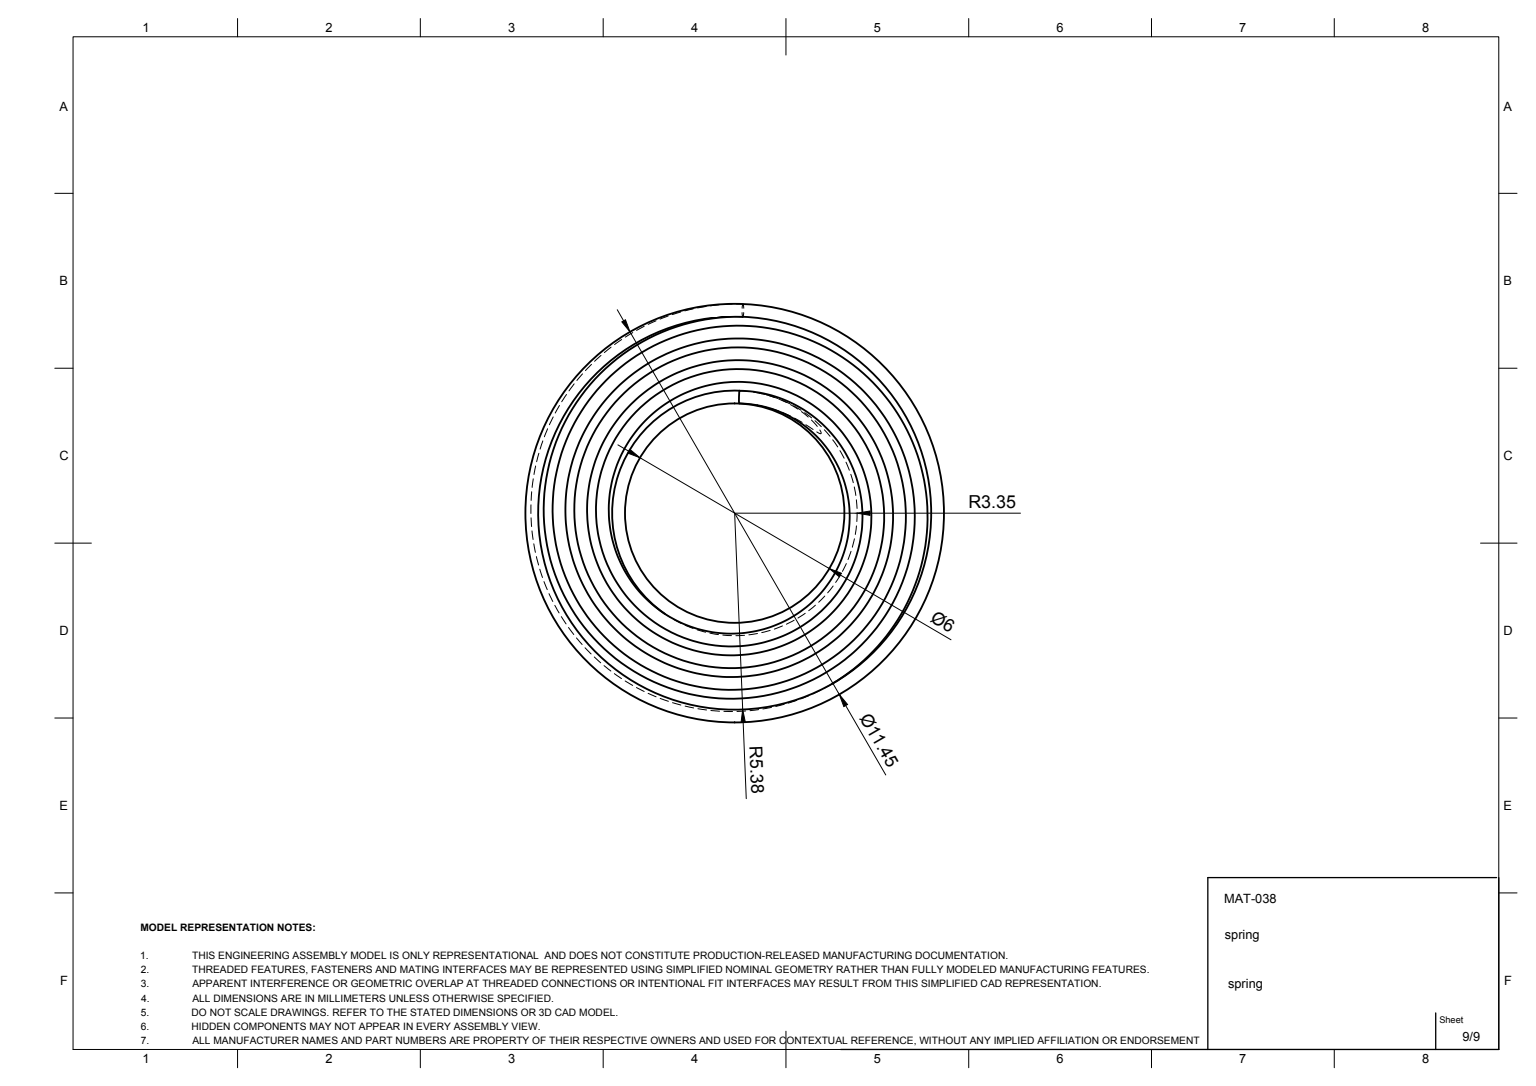
ISO-10303-21;
HEADER;
/* Generated by software containing ST-Developer
 * from STEP Tools, Inc. (www.steptools.com) 
 */

FILE_DESCRIPTION(
/* description */ ('STEP AP214'),
/* implementation_level */ '2;1');

FILE_NAME(
/* name */ 'Spring.step',
/* time_stamp */ '2026-11-14T21:32:33-08:00',
/* author */ (''),
/* organization */ (''),
/* preprocessor_version */ 'ST-DEVELOPER v20.2',
/* originating_system */ 'Autodesk Translation Framework v15.17.0.0',
/* authorisation */ '');

FILE_SCHEMA (('AUTOMOTIVE_DESIGN { 1 0 10303 214 3 1 1 }'));
ENDSEC;

DATA;
#10=MECHANICAL_DESIGN_GEOMETRIC_PRESENTATION_REPRESENTATION('',(#185,#186),#10551);
#47=(
BOUNDED_SURFACE()
B_SPLINE_SURFACE(3,3,((#8436,#8437,#8438,#8439,#8440,#8441,#8442,#8443,
#8444,#8445,#8446,#8447,#8448,#8449,#8450,#8451,#8452,#8453,#8454,#8455,
#8456,#8457,#8458,#8459,#8460,#8461,#8462,#8463,#8464,#8465,#8466,#8467,
#8468,#8469,#8470,#8471,#8472,#8473,#8474,#8475,#8476,#8477,#8478,#8479,
#8480,#8481,#8482,#8483,#8484,#8485,#8486,#8487,#8488,#8489,#8490,#8491,
#8492,#8493,#8494,#8495,#8496,#8497,#8498,#8499,#8500,#8501,#8502,#8503,
#8504,#8505,#8506,#8507,#8508,#8509,#8510,#8511,#8512,#8513,#8514,#8515,
#8516,#8517,#8518,#8519,#8520,#8521,#8522,#8523,#8524,#8525,#8526,#8527,
#8528,#8529,#8530,#8531,#8532,#8533,#8534,#8535,#8536,#8537,#8538,#8539,
#8540,#8541,#8542,#8543,#8544,#8545,#8546,#8547,#8548,#8549,#8550,#8551,
#8552,#8553,#8554,#8555,#8556,#8557,#8558,#8559,#8560,#8561,#8562,#8563,
#8564,#8565),(#8566,#8567,#8568,#8569,#8570,#8571,#8572,#8573,#8574,#8575,
#8576,#8577,#8578,#8579,#8580,#8581,#8582,#8583,#8584,#8585,#8586,#8587,
#8588,#8589,#8590,#8591,#8592,#8593,#8594,#8595,#8596,#8597,#8598,#8599,
#8600,#8601,#8602,#8603,#8604,#8605,#8606,#8607,#8608,#8609,#8610,#8611,
#8612,#8613,#8614,#8615,#8616,#8617,#8618,#8619,#8620,#8621,#8622,#8623,
#8624,#8625,#8626,#8627,#8628,#8629,#8630,#8631,#8632,#8633,#8634,#8635,
#8636,#8637,#8638,#8639,#8640,#8641,#8642,#8643,#8644,#8645,#8646,#8647,
#8648,#8649,#8650,#8651,#8652,#8653,#8654,#8655,#8656,#8657,#8658,#8659,
#8660,#8661,#8662,#8663,#8664,#8665,#8666,#8667,#8668,#8669,#8670,#8671,
#8672,#8673,#8674,#8675,#8676,#8677,#8678,#8679,#8680,#8681,#8682,#8683,
#8684,#8685,#8686,#8687,#8688,#8689,#8690,#8691,#8692,#8693,#8694,#8695),
(#8696,#8697,#8698,#8699,#8700,#8701,#8702,#8703,#8704,#8705,#8706,#8707,
#8708,#8709,#8710,#8711,#8712,#8713,#8714,#8715,#8716,#8717,#8718,#8719,
#8720,#8721,#8722,#8723,#8724,#8725,#8726,#8727,#8728,#8729,#8730,#8731,
#8732,#8733,#8734,#8735,#8736,#8737,#8738,#8739,#8740,#8741,#8742,#8743,
#8744,#8745,#8746,#8747,#8748,#8749,#8750,#8751,#8752,#8753,#8754,#8755,
#8756,#8757,#8758,#8759,#8760,#8761,#8762,#8763,#8764,#8765,#8766,#8767,
#8768,#8769,#8770,#8771,#8772,#8773,#8774,#8775,#8776,#8777,#8778,#8779,
#8780,#8781,#8782,#8783,#8784,#8785,#8786,#8787,#8788,#8789,#8790,#8791,
#8792,#8793,#8794,#8795,#8796,#8797,#8798,#8799,#8800,#8801,#8802,#8803,
#8804,#8805,#8806,#8807,#8808,#8809,#8810,#8811,#8812,#8813,#8814,#8815,
#8816,#8817,#8818,#8819,#8820,#8821,#8822,#8823,#8824,#8825),(#8826,#8827,
#8828,#8829,#8830,#8831,#8832,#8833,#8834,#8835,#8836,#8837,#8838,#8839,
#8840,#8841,#8842,#8843,#8844,#8845,#8846,#8847,#8848,#8849,#8850,#8851,
#8852,#8853,#8854,#8855,#8856,#8857,#8858,#8859,#8860,#8861,#8862,#8863,
#8864,#8865,#8866,#8867,#8868,#8869,#8870,#8871,#8872,#8873,#8874,#8875,
#8876,#8877,#8878,#8879,#8880,#8881,#8882,#8883,#8884,#8885,#8886,#8887,
#8888,#8889,#8890,#8891,#8892,#8893,#8894,#8895,#8896,#8897,#8898,#8899,
#8900,#8901,#8902,#8903,#8904,#8905,#8906,#8907,#8908,#8909,#8910,#8911,
#8912,#8913,#8914,#8915,#8916,#8917,#8918,#8919,#8920,#8921,#8922,#8923,
#8924,#8925,#8926,#8927,#8928,#8929,#8930,#8931,#8932,#8933,#8934,#8935,
#8936,#8937,#8938,#8939,#8940,#8941,#8942,#8943,#8944,#8945,#8946,#8947,
#8948,#8949,#8950,#8951,#8952,#8953,#8954,#8955),(#8956,#8957,#8958,#8959,
#8960,#8961,#8962,#8963,#8964,#8965,#8966,#8967,#8968,#8969,#8970,#8971,
#8972,#8973,#8974,#8975,#8976,#8977,#8978,#8979,#8980,#8981,#8982,#8983,
#8984,#8985,#8986,#8987,#8988,#8989,#8990,#8991,#8992,#8993,#8994,#8995,
#8996,#8997,#8998,#8999,#9000,#9001,#9002,#9003,#9004,#9005,#9006,#9007,
#9008,#9009,#9010,#9011,#9012,#9013,#9014,#9015,#9016,#9017,#9018,#9019,
#9020,#9021,#9022,#9023,#9024,#9025,#9026,#9027,#9028,#9029,#9030,#9031,
#9032,#9033,#9034,#9035,#9036,#9037,#9038,#9039,#9040,#9041,#9042,#9043,
#9044,#9045,#9046,#9047,#9048,#9049,#9050,#9051,#9052,#9053,#9054,#9055,
#9056,#9057,#9058,#9059,#9060,#9061,#9062,#9063,#9064,#9065,#9066,#9067,
#9068,#9069,#9070,#9071,#9072,#9073,#9074,#9075,#9076,#9077,#9078,#9079,
#9080,#9081,#9082,#9083,#9084,#9085),(#9086,#9087,#9088,#9089,#9090,#9091,
#9092,#9093,#9094,#9095,#9096,#9097,#9098,#9099,#9100,#9101,#9102,#9103,
#9104,#9105,#9106,#9107,#9108,#9109,#9110,#9111,#9112,#9113,#9114,#9115,
#9116,#9117,#9118,#9119,#9120,#9121,#9122,#9123,#9124,#9125,#9126,#9127,
#9128,#9129,#9130,#9131,#9132,#9133,#9134,#9135,#9136,#9137,#9138,#9139,
#9140,#9141,#9142,#9143,#9144,#9145,#9146,#9147,#9148,#9149,#9150,#9151,
#9152,#9153,#9154,#9155,#9156,#9157,#9158,#9159,#9160,#9161,#9162,#9163,
#9164,#9165,#9166,#9167,#9168,#9169,#9170,#9171,#9172,#9173,#9174,#9175,
#9176,#9177,#9178,#9179,#9180,#9181,#9182,#9183,#9184,#9185,#9186,#9187,
#9188,#9189,#9190,#9191,#9192,#9193,#9194,#9195,#9196,#9197,#9198,#9199,
#9200,#9201,#9202,#9203,#9204,#9205,#9206,#9207,#9208,#9209,#9210,#9211,
#9212,#9213,#9214,#9215),(#9216,#9217,#9218,#9219,#9220,#9221,#9222,#9223,
#9224,#9225,#9226,#9227,#9228,#9229,#9230,#9231,#9232,#9233,#9234,#9235,
#9236,#9237,#9238,#9239,#9240,#9241,#9242,#9243,#9244,#9245,#9246,#9247,
#9248,#9249,#9250,#9251,#9252,#9253,#9254,#9255,#9256,#9257,#9258,#9259,
#9260,#9261,#9262,#9263,#9264,#9265,#9266,#9267,#9268,#9269,#9270,#9271,
#9272,#9273,#9274,#9275,#9276,#9277,#9278,#9279,#9280,#9281,#9282,#9283,
#9284,#9285,#9286,#9287,#9288,#9289,#9290,#9291,#9292,#9293,#9294,#9295,
#9296,#9297,#9298,#9299,#9300,#9301,#9302,#9303,#9304,#9305,#9306,#9307,
#9308,#9309,#9310,#9311,#9312,#9313,#9314,#9315,#9316,#9317,#9318,#9319,
#9320,#9321,#9322,#9323,#9324,#9325,#9326,#9327,#9328,#9329,#9330,#9331,
#9332,#9333,#9334,#9335,#9336,#9337,#9338,#9339,#9340,#9341,#9342,#9343,
#9344,#9345)),.UNSPECIFIED.,.T.,.F.,.F.)
B_SPLINE_SURFACE_WITH_KNOTS((4,3,4),(4,2,2,2,2,2,2,2,2,2,2,2,2,2,2,2,2,
2,2,2,2,2,2,2,2,2,2,2,2,2,2,2,2,2,2,2,2,2,2,2,2,2,2,2,2,2,2,2,2,2,2,2,2,
2,2,2,2,2,2,2,2,2,2,2,4),(0.,0.5,1.),(-1.6716721247158E-5,0.015625,0.03125,
0.046875,0.0625,0.078125,0.09375,0.109375,0.125,0.140625,0.15625,0.171875,
0.1875,0.203125,0.21875,0.234375,0.25,0.265625,0.28125,0.296875,0.3125,
0.328125,0.34375,0.359375,0.375,0.390625,0.40625,0.421875,0.4375,0.453125,
0.46875,0.484375,0.5,0.515625,0.53125,0.546875,0.5625,0.578125,0.59375,
0.609375,0.625,0.640625,0.65625,0.671875,0.6875,0.703125,0.71875,0.734375,
0.75,0.765625,0.78125,0.796875,0.8125,0.828125,0.84375,0.859375,0.875,0.890625,
0.90625,0.921875,0.9375,0.953125,0.96875,0.984375,1.),.UNSPECIFIED.)
GEOMETRIC_REPRESENTATION_ITEM()
RATIONAL_B_SPLINE_SURFACE(((1.,1.,1.,1.,1.,1.,1.,1.,1.,1.,1.,1.,1.,1.,1.,
1.,1.,1.,1.,1.,1.,1.,1.,1.,1.,1.,1.,1.,1.,1.,1.,1.,1.,1.,1.,1.,1.,1.,1.,
1.,1.,1.,1.,1.,1.,1.,1.,1.,1.,1.,1.,1.,1.,1.,1.,1.,1.,1.,1.,1.,1.,1.,1.,
1.,1.,1.,1.,1.,1.,1.,1.,1.,1.,1.,1.,1.,1.,1.,1.,1.,1.,1.,1.,1.,1.,1.,1.,
1.,1.,1.,1.,1.,1.,1.,1.,1.,1.,1.,1.,1.,1.,1.,1.,1.,1.,1.,1.,1.,1.,1.,1.,
1.,1.,1.,1.,1.,1.,1.,1.,1.,1.,1.,1.,1.,1.,1.,1.,1.,1.,1.),(0.333333333333334,
0.333333333333333,0.333333333333333,0.333333333333333,0.333333333333333,
0.333333333333333,0.333333333333333,0.333333333333333,0.333333333333333,
0.333333333333333,0.333333333333333,0.333333333333333,0.333333333333333,
0.333333333333333,0.333333333333333,0.333333333333333,0.333333333333333,
0.333333333333333,0.333333333333333,0.333333333333333,0.333333333333333,
0.333333333333333,0.333333333333333,0.333333333333333,0.333333333333333,
0.333333333333333,0.333333333333333,0.333333333333333,0.333333333333333,
0.333333333333333,0.333333333333333,0.333333333333333,0.333333333333333,
0.333333333333333,0.333333333333333,0.333333333333333,0.333333333333333,
0.333333333333333,0.333333333333333,0.333333333333333,0.333333333333333,
0.333333333333333,0.333333333333333,0.333333333333333,0.333333333333333,
0.333333333333333,0.333333333333333,0.333333333333333,0.333333333333333,
0.333333333333333,0.333333333333333,0.333333333333333,0.333333333333333,
0.333333333333333,0.333333333333333,0.333333333333333,0.333333333333333,
0.333333333333333,0.333333333333333,0.333333333333333,0.333333333333333,
0.333333333333333,0.333333333333333,0.333333333333333,0.333333333333333,
0.333333333333333,0.333333333333333,0.333333333333333,0.333333333333333,
0.333333333333333,0.333333333333333,0.333333333333333,0.333333333333333,
0.333333333333333,0.333333333333333,0.333333333333333,0.333333333333333,
0.333333333333333,0.333333333333333,0.333333333333333,0.333333333333333,
0.333333333333333,0.333333333333333,0.333333333333333,0.333333333333333,
0.333333333333333,0.333333333333333,0.333333333333333,0.333333333333333,
0.333333333333333,0.333333333333333,0.333333333333333,0.333333333333333,
0.333333333333333,0.333333333333333,0.333333333333333,0.333333333333333,
0.333333333333333,0.333333333333333,0.333333333333333,0.333333333333333,
0.333333333333333,0.333333333333333,0.333333333333333,0.333333333333333,
0.333333333333333,0.333333333333333,0.333333333333333,0.333333333333333,
0.333333333333333,0.333333333333333,0.333333333333333,0.333333333333333,
0.333333333333333,0.333333333333333,0.333333333333333,0.333333333333333,
0.333333333333333,0.333333333333333,0.333333333333333,0.333333333333333,
0.333333333333333,0.333333333333333,0.333333333333333,0.333333333333333,
0.333333333333333,0.333333333333333,0.333333333333333,0.333333333333333,
0.333333333333333),(0.333333333333334,0.333333333333333,0.333333333333333,
0.333333333333333,0.333333333333333,0.333333333333333,0.333333333333333,
0.333333333333333,0.333333333333333,0.333333333333333,0.333333333333333,
0.333333333333333,0.333333333333333,0.333333333333333,0.333333333333333,
0.333333333333333,0.333333333333333,0.333333333333333,0.333333333333333,
0.333333333333333,0.333333333333333,0.333333333333333,0.333333333333333,
0.333333333333333,0.333333333333333,0.333333333333333,0.333333333333333,
0.333333333333333,0.333333333333333,0.333333333333333,0.333333333333333,
0.333333333333333,0.333333333333333,0.333333333333333,0.333333333333333,
0.333333333333333,0.333333333333333,0.333333333333333,0.333333333333333,
0.333333333333333,0.333333333333333,0.333333333333333,0.333333333333333,
0.333333333333333,0.333333333333333,0.333333333333333,0.333333333333333,
0.333333333333333,0.333333333333333,0.333333333333333,0.333333333333333,
0.333333333333333,0.333333333333333,0.333333333333333,0.333333333333333,
0.333333333333333,0.333333333333333,0.333333333333333,0.333333333333333,
0.333333333333333,0.333333333333333,0.333333333333333,0.333333333333333,
0.333333333333333,0.333333333333333,0.333333333333333,0.333333333333333,
0.333333333333333,0.333333333333333,0.333333333333333,0.333333333333333,
0.333333333333333,0.333333333333333,0.333333333333333,0.333333333333333,
0.333333333333333,0.333333333333333,0.333333333333333,0.333333333333333,
0.333333333333333,0.333333333333333,0.333333333333333,0.333333333333333,
0.333333333333333,0.333333333333333,0.333333333333333,0.333333333333333,
0.333333333333333,0.333333333333333,0.333333333333333,0.333333333333333,
0.333333333333333,0.333333333333333,0.333333333333333,0.333333333333333,
0.333333333333333,0.333333333333333,0.333333333333333,0.333333333333333,
0.333333333333333,0.333333333333333,0.333333333333333,0.333333333333333,
0.333333333333333,0.333333333333333,0.333333333333333,0.333333333333333,
0.333333333333333,0.333333333333333,0.333333333333333,0.333333333333333,
0.333333333333333,0.333333333333333,0.333333333333333,0.333333333333333,
0.333333333333333,0.333333333333333,0.333333333333333,0.333333333333333,
0.333333333333333,0.333333333333333,0.333333333333333,0.333333333333333,
0.333333333333333,0.333333333333333,0.333333333333333,0.333333333333333,
0.333333333333333,0.333333333333333,0.333333333333333),(1.,1.,1.,1.,1.,
1.,1.,1.,1.,1.,1.,1.,1.,1.,1.,1.,1.,1.,1.,1.,1.,1.,1.,1.,1.,1.,1.,1.,1.,
1.,1.,1.,1.,1.,1.,1.,1.,1.,1.,1.,1.,1.,1.,1.,1.,1.,1.,1.,1.,1.,1.,1.,1.,
1.,1.,1.,1.,1.,1.,1.,1.,1.,1.,1.,1.,1.,1.,1.,1.,1.,1.,1.,1.,1.,1.,1.,1.,
1.,1.,1.,1.,1.,1.,1.,1.,1.,1.,1.,1.,1.,1.,1.,1.,1.,1.,1.,1.,1.,1.,1.,1.,
1.,1.,1.,1.,1.,1.,1.,1.,1.,1.,1.,1.,1.,1.,1.,1.,1.,1.,1.,1.,1.,1.,1.,1.,
1.,1.,1.,1.,1.),(0.333333333333334,0.333333333333333,0.333333333333333,
0.333333333333333,0.333333333333333,0.333333333333333,0.333333333333333,
0.333333333333333,0.333333333333333,0.333333333333333,0.333333333333333,
0.333333333333333,0.333333333333333,0.333333333333333,0.333333333333333,
0.333333333333333,0.333333333333333,0.333333333333333,0.333333333333333,
0.333333333333333,0.333333333333333,0.333333333333333,0.333333333333333,
0.333333333333333,0.333333333333333,0.333333333333333,0.333333333333333,
0.333333333333333,0.333333333333333,0.333333333333333,0.333333333333333,
0.333333333333333,0.333333333333333,0.333333333333333,0.333333333333333,
0.333333333333333,0.333333333333333,0.333333333333333,0.333333333333333,
0.333333333333333,0.333333333333333,0.333333333333333,0.333333333333333,
0.333333333333333,0.333333333333333,0.333333333333333,0.333333333333333,
0.333333333333333,0.333333333333333,0.333333333333333,0.333333333333333,
0.333333333333333,0.333333333333333,0.333333333333333,0.333333333333333,
0.333333333333333,0.333333333333333,0.333333333333333,0.333333333333333,
0.333333333333333,0.333333333333333,0.333333333333333,0.333333333333333,
0.333333333333333,0.333333333333333,0.333333333333333,0.333333333333333,
0.333333333333333,0.333333333333333,0.333333333333333,0.333333333333333,
0.333333333333333,0.333333333333333,0.333333333333333,0.333333333333333,
0.333333333333333,0.333333333333333,0.333333333333333,0.333333333333333,
0.333333333333333,0.333333333333333,0.333333333333333,0.333333333333333,
0.333333333333333,0.333333333333333,0.333333333333333,0.333333333333333,
0.333333333333333,0.333333333333333,0.333333333333333,0.333333333333333,
0.333333333333333,0.333333333333333,0.333333333333333,0.333333333333333,
0.333333333333333,0.333333333333333,0.333333333333333,0.333333333333333,
0.333333333333333,0.333333333333333,0.333333333333333,0.333333333333333,
0.333333333333333,0.333333333333333,0.333333333333333,0.333333333333333,
0.333333333333333,0.333333333333333,0.333333333333333,0.333333333333333,
0.333333333333333,0.333333333333333,0.333333333333333,0.333333333333333,
0.333333333333333,0.333333333333333,0.333333333333333,0.333333333333333,
0.333333333333333,0.333333333333333,0.333333333333333,0.333333333333333,
0.333333333333333,0.333333333333333,0.333333333333333,0.333333333333333,
0.333333333333333,0.333333333333333,0.333333333333333),(0.333333333333334,
0.333333333333333,0.333333333333333,0.333333333333333,0.333333333333333,
0.333333333333333,0.333333333333333,0.333333333333333,0.333333333333333,
0.333333333333333,0.333333333333333,0.333333333333333,0.333333333333333,
0.333333333333333,0.333333333333333,0.333333333333333,0.333333333333333,
0.333333333333333,0.333333333333333,0.333333333333333,0.333333333333333,
0.333333333333333,0.333333333333333,0.333333333333333,0.333333333333333,
0.333333333333333,0.333333333333333,0.333333333333333,0.333333333333333,
0.333333333333333,0.333333333333333,0.333333333333333,0.333333333333333,
0.333333333333333,0.333333333333333,0.333333333333333,0.333333333333333,
0.333333333333333,0.333333333333333,0.333333333333333,0.333333333333333,
0.333333333333333,0.333333333333333,0.333333333333333,0.333333333333333,
0.333333333333333,0.333333333333333,0.333333333333333,0.333333333333333,
0.333333333333333,0.333333333333333,0.333333333333333,0.333333333333333,
0.333333333333333,0.333333333333333,0.333333333333333,0.333333333333333,
0.333333333333333,0.333333333333333,0.333333333333333,0.333333333333333,
0.333333333333333,0.333333333333333,0.333333333333333,0.333333333333333,
0.333333333333333,0.333333333333333,0.333333333333333,0.333333333333333,
0.333333333333333,0.333333333333333,0.333333333333333,0.333333333333333,
0.333333333333333,0.333333333333333,0.333333333333333,0.333333333333333,
0.333333333333333,0.333333333333333,0.333333333333333,0.333333333333333,
0.333333333333333,0.333333333333333,0.333333333333333,0.333333333333333,
0.333333333333333,0.333333333333333,0.333333333333333,0.333333333333333,
0.333333333333333,0.333333333333333,0.333333333333333,0.333333333333333,
0.333333333333333,0.333333333333333,0.333333333333333,0.333333333333333,
0.333333333333333,0.333333333333333,0.333333333333333,0.333333333333333,
0.333333333333333,0.333333333333333,0.333333333333333,0.333333333333333,
0.333333333333333,0.333333333333333,0.333333333333333,0.333333333333333,
0.333333333333333,0.333333333333333,0.333333333333333,0.333333333333333,
0.333333333333333,0.333333333333333,0.333333333333333,0.333333333333333,
0.333333333333333,0.333333333333333,0.333333333333333,0.333333333333333,
0.333333333333333,0.333333333333333,0.333333333333333,0.333333333333333,
0.333333333333333,0.333333333333333,0.333333333333333,0.333333333333333,
0.333333333333333),(1.,1.,1.,1.,1.,1.,1.,1.,1.,1.,1.,1.,1.,1.,1.,1.,1.,
1.,1.,1.,1.,1.,1.,1.,1.,1.,1.,1.,1.,1.,1.,1.,1.,1.,1.,1.,1.,1.,1.,1.,1.,
1.,1.,1.,1.,1.,1.,1.,1.,1.,1.,1.,1.,1.,1.,1.,1.,1.,1.,1.,1.,1.,1.,1.,1.,
1.,1.,1.,1.,1.,1.,1.,1.,1.,1.,1.,1.,1.,1.,1.,1.,1.,1.,1.,1.,1.,1.,1.,1.,
1.,1.,1.,1.,1.,1.,1.,1.,1.,1.,1.,1.,1.,1.,1.,1.,1.,1.,1.,1.,1.,1.,1.,1.,
1.,1.,1.,1.,1.,1.,1.,1.,1.,1.,1.,1.,1.,1.,1.,1.,1.)))
REPRESENTATION_ITEM('')
SURFACE()
);
#48=(
BOUNDED_SURFACE()
B_SPLINE_SURFACE(3,3,((#9609,#9610,#9611,#9612,#9613,#9614,#9615,#9616,
#9617,#9618,#9619,#9620,#9621,#9622,#9623,#9624,#9625,#9626,#9627,#9628,
#9629,#9630,#9631,#9632,#9633,#9634,#9635,#9636,#9637,#9638,#9639,#9640,
#9641,#9642,#9643,#9644,#9645,#9646,#9647,#9648,#9649,#9650,#9651,#9652,
#9653,#9654,#9655,#9656,#9657,#9658,#9659,#9660,#9661,#9662,#9663,#9664,
#9665,#9666,#9667,#9668,#9669,#9670,#9671,#9672,#9673,#9674,#9675,#9676,
#9677,#9678,#9679,#9680,#9681,#9682,#9683,#9684,#9685,#9686,#9687,#9688,
#9689,#9690,#9691,#9692,#9693,#9694,#9695,#9696,#9697,#9698,#9699,#9700,
#9701,#9702,#9703,#9704,#9705,#9706,#9707,#9708,#9709,#9710,#9711,#9712,
#9713,#9714,#9715,#9716,#9717,#9718,#9719,#9720,#9721,#9722,#9723,#9724,
#9725,#9726,#9727,#9728,#9729,#9730,#9731,#9732,#9733,#9734,#9735,#9736,
#9737,#9738),(#9739,#9740,#9741,#9742,#9743,#9744,#9745,#9746,#9747,#9748,
#9749,#9750,#9751,#9752,#9753,#9754,#9755,#9756,#9757,#9758,#9759,#9760,
#9761,#9762,#9763,#9764,#9765,#9766,#9767,#9768,#9769,#9770,#9771,#9772,
#9773,#9774,#9775,#9776,#9777,#9778,#9779,#9780,#9781,#9782,#9783,#9784,
#9785,#9786,#9787,#9788,#9789,#9790,#9791,#9792,#9793,#9794,#9795,#9796,
#9797,#9798,#9799,#9800,#9801,#9802,#9803,#9804,#9805,#9806,#9807,#9808,
#9809,#9810,#9811,#9812,#9813,#9814,#9815,#9816,#9817,#9818,#9819,#9820,
#9821,#9822,#9823,#9824,#9825,#9826,#9827,#9828,#9829,#9830,#9831,#9832,
#9833,#9834,#9835,#9836,#9837,#9838,#9839,#9840,#9841,#9842,#9843,#9844,
#9845,#9846,#9847,#9848,#9849,#9850,#9851,#9852,#9853,#9854,#9855,#9856,
#9857,#9858,#9859,#9860,#9861,#9862,#9863,#9864,#9865,#9866,#9867,#9868),
(#9869,#9870,#9871,#9872,#9873,#9874,#9875,#9876,#9877,#9878,#9879,#9880,
#9881,#9882,#9883,#9884,#9885,#9886,#9887,#9888,#9889,#9890,#9891,#9892,
#9893,#9894,#9895,#9896,#9897,#9898,#9899,#9900,#9901,#9902,#9903,#9904,
#9905,#9906,#9907,#9908,#9909,#9910,#9911,#9912,#9913,#9914,#9915,#9916,
#9917,#9918,#9919,#9920,#9921,#9922,#9923,#9924,#9925,#9926,#9927,#9928,
#9929,#9930,#9931,#9932,#9933,#9934,#9935,#9936,#9937,#9938,#9939,#9940,
#9941,#9942,#9943,#9944,#9945,#9946,#9947,#9948,#9949,#9950,#9951,#9952,
#9953,#9954,#9955,#9956,#9957,#9958,#9959,#9960,#9961,#9962,#9963,#9964,
#9965,#9966,#9967,#9968,#9969,#9970,#9971,#9972,#9973,#9974,#9975,#9976,
#9977,#9978,#9979,#9980,#9981,#9982,#9983,#9984,#9985,#9986,#9987,#9988,
#9989,#9990,#9991,#9992,#9993,#9994,#9995,#9996,#9997,#9998),(#9999,#10000,
#10001,#10002,#10003,#10004,#10005,#10006,#10007,#10008,#10009,#10010,#10011,
#10012,#10013,#10014,#10015,#10016,#10017,#10018,#10019,#10020,#10021,#10022,
#10023,#10024,#10025,#10026,#10027,#10028,#10029,#10030,#10031,#10032,#10033,
#10034,#10035,#10036,#10037,#10038,#10039,#10040,#10041,#10042,#10043,#10044,
#10045,#10046,#10047,#10048,#10049,#10050,#10051,#10052,#10053,#10054,#10055,
#10056,#10057,#10058,#10059,#10060,#10061,#10062,#10063,#10064,#10065,#10066,
#10067,#10068,#10069,#10070,#10071,#10072,#10073,#10074,#10075,#10076,#10077,
#10078,#10079,#10080,#10081,#10082,#10083,#10084,#10085,#10086,#10087,#10088,
#10089,#10090,#10091,#10092,#10093,#10094,#10095,#10096,#10097,#10098,#10099,
#10100,#10101,#10102,#10103,#10104,#10105,#10106,#10107,#10108,#10109,#10110,
#10111,#10112,#10113,#10114,#10115,#10116,#10117,#10118,#10119,#10120,#10121,
#10122,#10123,#10124,#10125,#10126,#10127,#10128),(#10129,#10130,#10131,
#10132,#10133,#10134,#10135,#10136,#10137,#10138,#10139,#10140,#10141,#10142,
#10143,#10144,#10145,#10146,#10147,#10148,#10149,#10150,#10151,#10152,#10153,
#10154,#10155,#10156,#10157,#10158,#10159,#10160,#10161,#10162,#10163,#10164,
#10165,#10166,#10167,#10168,#10169,#10170,#10171,#10172,#10173,#10174,#10175,
#10176,#10177,#10178,#10179,#10180,#10181,#10182,#10183,#10184,#10185,#10186,
#10187,#10188,#10189,#10190,#10191,#10192,#10193,#10194,#10195,#10196,#10197,
#10198,#10199,#10200,#10201,#10202,#10203,#10204,#10205,#10206,#10207,#10208,
#10209,#10210,#10211,#10212,#10213,#10214,#10215,#10216,#10217,#10218,#10219,
#10220,#10221,#10222,#10223,#10224,#10225,#10226,#10227,#10228,#10229,#10230,
#10231,#10232,#10233,#10234,#10235,#10236,#10237,#10238,#10239,#10240,#10241,
#10242,#10243,#10244,#10245,#10246,#10247,#10248,#10249,#10250,#10251,#10252,
#10253,#10254,#10255,#10256,#10257,#10258),(#10259,#10260,#10261,#10262,
#10263,#10264,#10265,#10266,#10267,#10268,#10269,#10270,#10271,#10272,#10273,
#10274,#10275,#10276,#10277,#10278,#10279,#10280,#10281,#10282,#10283,#10284,
#10285,#10286,#10287,#10288,#10289,#10290,#10291,#10292,#10293,#10294,#10295,
#10296,#10297,#10298,#10299,#10300,#10301,#10302,#10303,#10304,#10305,#10306,
#10307,#10308,#10309,#10310,#10311,#10312,#10313,#10314,#10315,#10316,#10317,
#10318,#10319,#10320,#10321,#10322,#10323,#10324,#10325,#10326,#10327,#10328,
#10329,#10330,#10331,#10332,#10333,#10334,#10335,#10336,#10337,#10338,#10339,
#10340,#10341,#10342,#10343,#10344,#10345,#10346,#10347,#10348,#10349,#10350,
#10351,#10352,#10353,#10354,#10355,#10356,#10357,#10358,#10359,#10360,#10361,
#10362,#10363,#10364,#10365,#10366,#10367,#10368,#10369,#10370,#10371,#10372,
#10373,#10374,#10375,#10376,#10377,#10378,#10379,#10380,#10381,#10382,#10383,
#10384,#10385,#10386,#10387,#10388),(#10389,#10390,#10391,#10392,#10393,
#10394,#10395,#10396,#10397,#10398,#10399,#10400,#10401,#10402,#10403,#10404,
#10405,#10406,#10407,#10408,#10409,#10410,#10411,#10412,#10413,#10414,#10415,
#10416,#10417,#10418,#10419,#10420,#10421,#10422,#10423,#10424,#10425,#10426,
#10427,#10428,#10429,#10430,#10431,#10432,#10433,#10434,#10435,#10436,#10437,
#10438,#10439,#10440,#10441,#10442,#10443,#10444,#10445,#10446,#10447,#10448,
#10449,#10450,#10451,#10452,#10453,#10454,#10455,#10456,#10457,#10458,#10459,
#10460,#10461,#10462,#10463,#10464,#10465,#10466,#10467,#10468,#10469,#10470,
#10471,#10472,#10473,#10474,#10475,#10476,#10477,#10478,#10479,#10480,#10481,
#10482,#10483,#10484,#10485,#10486,#10487,#10488,#10489,#10490,#10491,#10492,
#10493,#10494,#10495,#10496,#10497,#10498,#10499,#10500,#10501,#10502,#10503,
#10504,#10505,#10506,#10507,#10508,#10509,#10510,#10511,#10512,#10513,#10514,
#10515,#10516,#10517,#10518)),.UNSPECIFIED.,.T.,.F.,.F.)
B_SPLINE_SURFACE_WITH_KNOTS((4,3,4),(4,2,2,2,2,2,2,2,2,2,2,2,2,2,2,2,2,
2,2,2,2,2,2,2,2,2,2,2,2,2,2,2,2,2,2,2,2,2,2,2,2,2,2,2,2,2,2,2,2,2,2,2,2,
2,2,2,2,2,2,2,2,2,2,2,4),(0.,0.5,1.),(0.,0.015625,0.03125,0.046875,0.0625,
0.078125,0.09375,0.109375,0.125,0.140625,0.15625,0.171875,0.1875,0.203125,
0.21875,0.234375,0.25,0.265625,0.28125,0.296875,0.3125,0.328125,0.34375,
0.359375,0.375,0.390625,0.40625,0.421875,0.4375,0.453125,0.46875,0.484375,
0.5,0.515625,0.53125,0.546875,0.5625,0.578125,0.59375,0.609375,0.625,0.640625,
0.65625,0.671875,0.6875,0.703125,0.71875,0.734375,0.75,0.765625,0.78125,
0.796875,0.8125,0.828125,0.84375,0.859375,0.875,0.890625,0.90625,0.921875,
0.9375,0.953125,0.96875,0.984375,1.),.UNSPECIFIED.)
GEOMETRIC_REPRESENTATION_ITEM()
RATIONAL_B_SPLINE_SURFACE(((1.,1.,1.,1.,1.,1.,1.,1.,1.,1.,1.,1.,1.,1.,1.,
1.,1.,1.,1.,1.,1.,1.,1.,1.,1.,1.,1.,1.,1.,1.,1.,1.,1.,1.,1.,1.,1.,1.,1.,
1.,1.,1.,1.,1.,1.,1.,1.,1.,1.,1.,1.,1.,1.,1.,1.,1.,1.,1.,1.,1.,1.,1.,1.,
1.,1.,1.,1.,1.,1.,1.,1.,1.,1.,1.,1.,1.,1.,1.,1.,1.,1.,1.,1.,1.,1.,1.,1.,
1.,1.,1.,1.,1.,1.,1.,1.,1.,1.,1.,1.,1.,1.,1.,1.,1.,1.,1.,1.,1.,1.,1.,1.,
1.,1.,1.,1.,1.,1.,1.,1.,1.,1.,1.,1.,1.,1.,1.,1.,1.,1.,1.),(0.333333333333333,
0.333333333333333,0.333333333333333,0.333333333333333,0.333333333333333,
0.333333333333333,0.333333333333333,0.333333333333333,0.333333333333333,
0.333333333333333,0.333333333333333,0.333333333333333,0.333333333333333,
0.333333333333333,0.333333333333333,0.333333333333333,0.333333333333333,
0.333333333333333,0.333333333333333,0.333333333333333,0.333333333333333,
0.333333333333333,0.333333333333333,0.333333333333333,0.333333333333333,
0.333333333333333,0.333333333333333,0.333333333333333,0.333333333333333,
0.333333333333333,0.333333333333333,0.333333333333333,0.333333333333333,
0.333333333333333,0.333333333333333,0.333333333333333,0.333333333333333,
0.333333333333333,0.333333333333333,0.333333333333333,0.333333333333333,
0.333333333333333,0.333333333333333,0.333333333333333,0.333333333333333,
0.333333333333333,0.333333333333333,0.333333333333333,0.333333333333333,
0.333333333333333,0.333333333333333,0.333333333333333,0.333333333333333,
0.333333333333333,0.333333333333333,0.333333333333333,0.333333333333333,
0.333333333333333,0.333333333333333,0.333333333333333,0.333333333333333,
0.333333333333333,0.333333333333333,0.333333333333333,0.333333333333333,
0.333333333333333,0.333333333333333,0.333333333333333,0.333333333333333,
0.333333333333333,0.333333333333333,0.333333333333333,0.333333333333333,
0.333333333333333,0.333333333333333,0.333333333333333,0.333333333333333,
0.333333333333333,0.333333333333333,0.333333333333333,0.333333333333333,
0.333333333333333,0.333333333333333,0.333333333333333,0.333333333333333,
0.333333333333333,0.333333333333333,0.333333333333333,0.333333333333333,
0.333333333333333,0.333333333333333,0.333333333333333,0.333333333333333,
0.333333333333333,0.333333333333333,0.333333333333333,0.333333333333333,
0.333333333333333,0.333333333333333,0.333333333333333,0.333333333333333,
0.333333333333333,0.333333333333333,0.333333333333333,0.333333333333333,
0.333333333333333,0.333333333333333,0.333333333333333,0.333333333333333,
0.333333333333333,0.333333333333333,0.333333333333333,0.333333333333333,
0.333333333333333,0.333333333333333,0.333333333333333,0.333333333333333,
0.333333333333333,0.333333333333333,0.333333333333333,0.333333333333333,
0.333333333333333,0.333333333333333,0.333333333333333,0.333333333333333,
0.333333333333333,0.333333333333333,0.333333333333333,0.333333333333333,
0.333333333333333),(0.333333333333333,0.333333333333333,0.333333333333333,
0.333333333333333,0.333333333333333,0.333333333333333,0.333333333333333,
0.333333333333333,0.333333333333333,0.333333333333333,0.333333333333333,
0.333333333333333,0.333333333333333,0.333333333333333,0.333333333333333,
0.333333333333333,0.333333333333333,0.333333333333333,0.333333333333333,
0.333333333333333,0.333333333333333,0.333333333333333,0.333333333333333,
0.333333333333333,0.333333333333333,0.333333333333333,0.333333333333333,
0.333333333333333,0.333333333333333,0.333333333333333,0.333333333333333,
0.333333333333333,0.333333333333333,0.333333333333333,0.333333333333333,
0.333333333333333,0.333333333333333,0.333333333333333,0.333333333333333,
0.333333333333333,0.333333333333333,0.333333333333333,0.333333333333333,
0.333333333333333,0.333333333333333,0.333333333333333,0.333333333333333,
0.333333333333333,0.333333333333333,0.333333333333333,0.333333333333333,
0.333333333333333,0.333333333333333,0.333333333333333,0.333333333333333,
0.333333333333333,0.333333333333333,0.333333333333333,0.333333333333333,
0.333333333333333,0.333333333333333,0.333333333333333,0.333333333333333,
0.333333333333333,0.333333333333333,0.333333333333333,0.333333333333333,
0.333333333333333,0.333333333333333,0.333333333333333,0.333333333333333,
0.333333333333333,0.333333333333333,0.333333333333333,0.333333333333333,
0.333333333333333,0.333333333333333,0.333333333333333,0.333333333333333,
0.333333333333333,0.333333333333333,0.333333333333333,0.333333333333333,
0.333333333333333,0.333333333333333,0.333333333333333,0.333333333333333,
0.333333333333333,0.333333333333333,0.333333333333333,0.333333333333333,
0.333333333333333,0.333333333333333,0.333333333333333,0.333333333333333,
0.333333333333333,0.333333333333333,0.333333333333333,0.333333333333333,
0.333333333333333,0.333333333333333,0.333333333333333,0.333333333333333,
0.333333333333333,0.333333333333333,0.333333333333333,0.333333333333333,
0.333333333333333,0.333333333333333,0.333333333333333,0.333333333333333,
0.333333333333333,0.333333333333333,0.333333333333333,0.333333333333333,
0.333333333333333,0.333333333333333,0.333333333333333,0.333333333333333,
0.333333333333333,0.333333333333333,0.333333333333333,0.333333333333333,
0.333333333333333,0.333333333333333,0.333333333333333,0.333333333333333,
0.333333333333333,0.333333333333333,0.333333333333333),(1.,1.,1.,1.,1.,
1.,1.,1.,1.,1.,1.,1.,1.,1.,1.,1.,1.,1.,1.,1.,1.,1.,1.,1.,1.,1.,1.,1.,1.,
1.,1.,1.,1.,1.,1.,1.,1.,1.,1.,1.,1.,1.,1.,1.,1.,1.,1.,1.,1.,1.,1.,1.,1.,
1.,1.,1.,1.,1.,1.,1.,1.,1.,1.,1.,1.,1.,1.,1.,1.,1.,1.,1.,1.,1.,1.,1.,1.,
1.,1.,1.,1.,1.,1.,1.,1.,1.,1.,1.,1.,1.,1.,1.,1.,1.,1.,1.,1.,1.,1.,1.,1.,
1.,1.,1.,1.,1.,1.,1.,1.,1.,1.,1.,1.,1.,1.,1.,1.,1.,1.,1.,1.,1.,1.,1.,1.,
1.,1.,1.,1.,1.),(0.333333333333333,0.333333333333333,0.333333333333333,
0.333333333333333,0.333333333333333,0.333333333333333,0.333333333333333,
0.333333333333333,0.333333333333333,0.333333333333333,0.333333333333333,
0.333333333333333,0.333333333333333,0.333333333333333,0.333333333333333,
0.333333333333333,0.333333333333333,0.333333333333333,0.333333333333333,
0.333333333333333,0.333333333333333,0.333333333333333,0.333333333333333,
0.333333333333333,0.333333333333333,0.333333333333333,0.333333333333333,
0.333333333333333,0.333333333333333,0.333333333333333,0.333333333333333,
0.333333333333333,0.333333333333333,0.333333333333333,0.333333333333333,
0.333333333333333,0.333333333333333,0.333333333333333,0.333333333333333,
0.333333333333333,0.333333333333333,0.333333333333333,0.333333333333333,
0.333333333333333,0.333333333333333,0.333333333333333,0.333333333333333,
0.333333333333333,0.333333333333333,0.333333333333333,0.333333333333333,
0.333333333333333,0.333333333333333,0.333333333333333,0.333333333333333,
0.333333333333333,0.333333333333333,0.333333333333333,0.333333333333333,
0.333333333333333,0.333333333333333,0.333333333333333,0.333333333333333,
0.333333333333333,0.333333333333333,0.333333333333333,0.333333333333333,
0.333333333333333,0.333333333333333,0.333333333333333,0.333333333333333,
0.333333333333333,0.333333333333333,0.333333333333333,0.333333333333333,
0.333333333333333,0.333333333333333,0.333333333333333,0.333333333333333,
0.333333333333333,0.333333333333333,0.333333333333333,0.333333333333333,
0.333333333333333,0.333333333333333,0.333333333333333,0.333333333333333,
0.333333333333333,0.333333333333333,0.333333333333333,0.333333333333333,
0.333333333333333,0.333333333333333,0.333333333333333,0.333333333333333,
0.333333333333333,0.333333333333333,0.333333333333333,0.333333333333333,
0.333333333333333,0.333333333333333,0.333333333333333,0.333333333333333,
0.333333333333333,0.333333333333333,0.333333333333333,0.333333333333333,
0.333333333333333,0.333333333333333,0.333333333333333,0.333333333333333,
0.333333333333333,0.333333333333333,0.333333333333333,0.333333333333333,
0.333333333333333,0.333333333333333,0.333333333333333,0.333333333333333,
0.333333333333333,0.333333333333333,0.333333333333333,0.333333333333333,
0.333333333333333,0.333333333333333,0.333333333333333,0.333333333333333,
0.333333333333333,0.333333333333333,0.333333333333333),(0.333333333333333,
0.333333333333333,0.333333333333333,0.333333333333333,0.333333333333333,
0.333333333333333,0.333333333333333,0.333333333333333,0.333333333333333,
0.333333333333333,0.333333333333333,0.333333333333333,0.333333333333333,
0.333333333333333,0.333333333333333,0.333333333333333,0.333333333333333,
0.333333333333333,0.333333333333333,0.333333333333333,0.333333333333333,
0.333333333333333,0.333333333333333,0.333333333333333,0.333333333333333,
0.333333333333333,0.333333333333333,0.333333333333333,0.333333333333333,
0.333333333333333,0.333333333333333,0.333333333333333,0.333333333333333,
0.333333333333333,0.333333333333333,0.333333333333333,0.333333333333333,
0.333333333333333,0.333333333333333,0.333333333333333,0.333333333333333,
0.333333333333333,0.333333333333333,0.333333333333333,0.333333333333333,
0.333333333333333,0.333333333333333,0.333333333333333,0.333333333333333,
0.333333333333333,0.333333333333333,0.333333333333333,0.333333333333333,
0.333333333333333,0.333333333333333,0.333333333333333,0.333333333333333,
0.333333333333333,0.333333333333333,0.333333333333333,0.333333333333333,
0.333333333333333,0.333333333333333,0.333333333333333,0.333333333333333,
0.333333333333333,0.333333333333333,0.333333333333333,0.333333333333333,
0.333333333333333,0.333333333333333,0.333333333333333,0.333333333333333,
0.333333333333333,0.333333333333333,0.333333333333333,0.333333333333333,
0.333333333333333,0.333333333333333,0.333333333333333,0.333333333333333,
0.333333333333333,0.333333333333333,0.333333333333333,0.333333333333333,
0.333333333333333,0.333333333333333,0.333333333333333,0.333333333333333,
0.333333333333333,0.333333333333333,0.333333333333333,0.333333333333333,
0.333333333333333,0.333333333333333,0.333333333333333,0.333333333333333,
0.333333333333333,0.333333333333333,0.333333333333333,0.333333333333333,
0.333333333333333,0.333333333333333,0.333333333333333,0.333333333333333,
0.333333333333333,0.333333333333333,0.333333333333333,0.333333333333333,
0.333333333333333,0.333333333333333,0.333333333333333,0.333333333333333,
0.333333333333333,0.333333333333333,0.333333333333333,0.333333333333333,
0.333333333333333,0.333333333333333,0.333333333333333,0.333333333333333,
0.333333333333333,0.333333333333333,0.333333333333333,0.333333333333333,
0.333333333333333,0.333333333333333,0.333333333333333,0.333333333333333,
0.333333333333333),(1.,1.,1.,1.,1.,1.,1.,1.,1.,1.,1.,1.,1.,1.,1.,1.,1.,
1.,1.,1.,1.,1.,1.,1.,1.,1.,1.,1.,1.,1.,1.,1.,1.,1.,1.,1.,1.,1.,1.,1.,1.,
1.,1.,1.,1.,1.,1.,1.,1.,1.,1.,1.,1.,1.,1.,1.,1.,1.,1.,1.,1.,1.,1.,1.,1.,
1.,1.,1.,1.,1.,1.,1.,1.,1.,1.,1.,1.,1.,1.,1.,1.,1.,1.,1.,1.,1.,1.,1.,1.,
1.,1.,1.,1.,1.,1.,1.,1.,1.,1.,1.,1.,1.,1.,1.,1.,1.,1.,1.,1.,1.,1.,1.,1.,
1.,1.,1.,1.,1.,1.,1.,1.,1.,1.,1.,1.,1.,1.,1.,1.,1.)))
REPRESENTATION_ITEM('')
SURFACE()
);
#49=ELLIPSE('',#4023,0.175430953951623,0.175001932698577);
#133=TOROIDAL_SURFACE('',#4017,5.55,0.175);
#134=TOROIDAL_SURFACE('',#4020,3.17573472959676,0.175);
#150=B_SPLINE_CURVE_WITH_KNOTS('',3,(#8379,#8380,#8381,#8382,#8383,#8384,
#8385,#8386),.UNSPECIFIED.,.F.,.F.,(4,2,2,4),(-0.000183878052419735,0.,
0.00168136886964635,0.00357997544050363),.UNSPECIFIED.);
#151=B_SPLINE_CURVE_WITH_KNOTS('',3,(#8388,#8389,#8390,#8391,#8392,#8393,
#8394,#8395,#8396,#8397,#8398,#8399,#8400,#8401,#8402,#8403,#8404,#8405,
#8406,#8407,#8408,#8409,#8410,#8411,#8412,#8413,#8414,#8415,#8416,#8417,
#8418,#8419,#8420,#8421,#8422,#8423),.UNSPECIFIED.,.F.,.F.,(4,2,2,2,2,2,
2,2,2,2,2,2,2,2,2,2,2,4),(-0.574674927918272,-0.571952286676393,-0.508824986264653,
-0.441235232795549,-0.327513816563257,-0.270706788955357,-0.257131961119942,
-0.253114953696847,-0.25068545375721,-0.248656048688706,-0.24640797600825,
-0.242733690405177,-0.23450108496833,-0.210223290532083,-0.0958268045063037,
-0.0460408693976727,-0.0223119527990917,-9.99999999917733E-7),
 .UNSPECIFIED.);
#152=B_SPLINE_CURVE_WITH_KNOTS('',3,(#8425,#8426,#8427,#8428,#8429,#8430,
#8431,#8432,#8433,#8434),.UNSPECIFIED.,.F.,.F.,(4,3,3,4),(0.00457726855862458,
0.00480753339462812,0.0050279498472682,0.00507749417619398),
 .UNSPECIFIED.);
#153=B_SPLINE_CURVE_WITH_KNOTS('',3,(#9347,#9348,#9349,#9350,#9351,#9352,
#9353,#9354,#9355,#9356,#9357,#9358,#9359,#9360,#9361,#9362,#9363,#9364,
#9365,#9366,#9367,#9368,#9369,#9370,#9371,#9372,#9373,#9374,#9375,#9376,
#9377,#9378,#9379,#9380,#9381,#9382,#9383,#9384,#9385,#9386,#9387,#9388,
#9389,#9390,#9391,#9392,#9393,#9394,#9395,#9396,#9397,#9398,#9399,#9400,
#9401,#9402,#9403,#9404,#9405,#9406,#9407,#9408,#9409,#9410,#9411,#9412,
#9413,#9414,#9415,#9416,#9417,#9418,#9419,#9420,#9421,#9422,#9423,#9424,
#9425,#9426,#9427,#9428,#9429,#9430,#9431,#9432,#9433,#9434,#9435,#9436,
#9437,#9438,#9439,#9440,#9441,#9442,#9443,#9444,#9445,#9446,#9447,#9448,
#9449,#9450,#9451,#9452,#9453,#9454,#9455,#9456,#9457,#9458,#9459,#9460,
#9461,#9462,#9463,#9464,#9465,#9466,#9467,#9468,#9469,#9470,#9471,#9472,
#9473,#9474,#9475,#9476),.UNSPECIFIED.,.F.,.F.,(4,2,2,2,2,2,2,2,2,2,2,2,
2,2,2,2,2,2,2,2,2,2,2,2,2,2,2,2,2,2,2,2,2,2,2,2,2,2,2,2,2,2,2,2,2,2,2,2,
2,2,2,2,2,2,2,2,2,2,2,2,2,2,2,2,4),(0.00652527768169836,0.015625,0.03125,
0.046875,0.0625,0.078125,0.09375,0.109375,0.125,0.140625,0.15625,0.171875,
0.1875,0.203125,0.21875,0.234375,0.25,0.265625,0.28125,0.296875,0.3125,
0.328125,0.34375,0.359375,0.375,0.390625,0.40625,0.421875,0.4375,0.453125,
0.46875,0.484375,0.5,0.515625,0.53125,0.546875,0.5625,0.578125,0.59375,
0.609375,0.625,0.640625,0.65625,0.671875,0.6875,0.703125,0.71875,0.734375,
0.75,0.765625,0.78125,0.796875,0.8125,0.828125,0.84375,0.859375,0.875,0.890625,
0.90625,0.921875,0.9375,0.953125,0.96875,0.984375,1.),.UNSPECIFIED.);
#154=B_SPLINE_CURVE_WITH_KNOTS('',3,(#9479,#9480,#9481,#9482,#9483,#9484,
#9485,#9486,#9487,#9488,#9489,#9490,#9491,#9492,#9493,#9494,#9495,#9496,
#9497,#9498,#9499,#9500,#9501,#9502,#9503,#9504,#9505,#9506,#9507,#9508,
#9509,#9510,#9511,#9512,#9513,#9514,#9515,#9516,#9517,#9518,#9519,#9520,
#9521,#9522,#9523,#9524,#9525,#9526,#9527,#9528,#9529,#9530,#9531,#9532,
#9533,#9534,#9535,#9536,#9537,#9538,#9539,#9540,#9541,#9542,#9543,#9544,
#9545,#9546,#9547,#9548,#9549,#9550,#9551,#9552,#9553,#9554,#9555,#9556,
#9557,#9558,#9559,#9560,#9561,#9562,#9563,#9564,#9565,#9566,#9567,#9568,
#9569,#9570,#9571,#9572,#9573,#9574,#9575,#9576,#9577,#9578,#9579,#9580,
#9581,#9582,#9583,#9584,#9585,#9586,#9587,#9588,#9589,#9590,#9591,#9592,
#9593,#9594,#9595,#9596,#9597,#9598,#9599,#9600,#9601,#9602,#9603,#9604,
#9605,#9606,#9607,#9608),.UNSPECIFIED.,.F.,.F.,(4,2,2,2,2,2,2,2,2,2,2,2,
2,2,2,2,2,2,2,2,2,2,2,2,2,2,2,2,2,2,2,2,2,2,2,2,2,2,2,2,2,2,2,2,2,2,2,2,
2,2,2,2,2,2,2,2,2,2,2,2,2,2,2,2,4),(3.07557452178047E-5,0.015625,0.03125,
0.046875,0.0625,0.078125,0.09375,0.109375,0.125,0.140625,0.15625,0.171875,
0.1875,0.203125,0.21875,0.234375,0.25,0.265625,0.28125,0.296875,0.3125,
0.328125,0.34375,0.359375,0.375,0.390625,0.40625,0.421875,0.4375,0.453125,
0.46875,0.484375,0.5,0.515625,0.53125,0.546875,0.5625,0.578125,0.59375,
0.609375,0.625,0.640625,0.65625,0.671875,0.6875,0.703125,0.71875,0.734375,
0.75,0.765625,0.78125,0.796875,0.8125,0.828125,0.84375,0.859375,0.875,0.890625,
0.90625,0.921875,0.9375,0.953125,0.96875,0.984375,1.),.UNSPECIFIED.);
#167=SHAPE_REPRESENTATION_RELATIONSHIP('SRR','None',#10594,#176);
#176=ADVANCED_BREP_SHAPE_REPRESENTATION('',(#195,#196),#10550);
#185=STYLED_ITEM('',(#10645),#195);
#186=STYLED_ITEM('',(#10645),#196);
#195=MANIFOLD_SOLID_BREP('Body1',#3434);
#196=MANIFOLD_SOLID_BREP('Body2',#3435);
#223=FACE_BOUND('',#757,.T.);
#293=PLANE('',#4026);
#509=FACE_OUTER_BOUND('',#755,.T.);
#510=FACE_OUTER_BOUND('',#756,.T.);
#511=FACE_OUTER_BOUND('',#758,.T.);
#512=FACE_OUTER_BOUND('',#759,.T.);
#513=FACE_OUTER_BOUND('',#760,.T.);
#755=EDGE_LOOP('',(#3126,#3127,#3128,#3129));
#756=EDGE_LOOP('',(#3130,#3131,#3132,#3133));
#757=EDGE_LOOP('',(#3134,#3135,#3136,#3137));
#758=EDGE_LOOP('',(#3138,#3139,#3140,#3141,#3142));
#759=EDGE_LOOP('',(#3143,#3144,#3145,#3146,#3147));
#760=EDGE_LOOP('',(#3148,#3149));
#1415=CIRCLE('',#4018,0.175);
#1416=CIRCLE('',#4019,5.375);
#1417=CIRCLE('',#4021,0.175);
#1418=CIRCLE('',#4022,3.00073472959676);
#1419=CIRCLE('',#4024,0.175);
#1420=CIRCLE('',#4025,0.175);
#1699=VERTEX_POINT('',#8370);
#1700=VERTEX_POINT('',#8374);
#1701=VERTEX_POINT('',#8377);
#1702=VERTEX_POINT('',#8378);
#1703=VERTEX_POINT('',#8387);
#1704=VERTEX_POINT('',#8424);
#1705=VERTEX_POINT('',#9346);
#1706=VERTEX_POINT('',#9477);
#2176=EDGE_CURVE('',#1699,#1699,#1415,.T.);
#2177=EDGE_CURVE('',#1699,#1699,#1416,.T.);
#2178=EDGE_CURVE('',#1700,#1700,#1417,.T.);
#2179=EDGE_CURVE('',#1700,#1700,#1418,.T.);
#2180=EDGE_CURVE('',#1701,#1702,#150,.F.);
#2181=EDGE_CURVE('',#1702,#1703,#151,.T.);
#2182=EDGE_CURVE('',#1703,#1704,#152,.T.);
#2183=EDGE_CURVE('',#1704,#1701,#49,.T.);
#2184=EDGE_CURVE('',#1703,#1705,#153,.T.);
#2185=EDGE_CURVE('',#1705,#1706,#1419,.T.);
#2186=EDGE_CURVE('',#1701,#1706,#154,.T.);
#2187=EDGE_CURVE('',#1706,#1705,#1420,.T.);
#3126=ORIENTED_EDGE('',*,*,#2176,.F.);
#3127=ORIENTED_EDGE('',*,*,#2177,.T.);
#3128=ORIENTED_EDGE('',*,*,#2176,.T.);
#3129=ORIENTED_EDGE('',*,*,#2177,.F.);
#3130=ORIENTED_EDGE('',*,*,#2178,.F.);
#3131=ORIENTED_EDGE('',*,*,#2179,.T.);
#3132=ORIENTED_EDGE('',*,*,#2178,.T.);
#3133=ORIENTED_EDGE('',*,*,#2179,.F.);
#3134=ORIENTED_EDGE('',*,*,#2180,.T.);
#3135=ORIENTED_EDGE('',*,*,#2181,.T.);
#3136=ORIENTED_EDGE('',*,*,#2182,.T.);
#3137=ORIENTED_EDGE('',*,*,#2183,.T.);
#3138=ORIENTED_EDGE('',*,*,#2182,.F.);
#3139=ORIENTED_EDGE('',*,*,#2184,.T.);
#3140=ORIENTED_EDGE('',*,*,#2185,.T.);
#3141=ORIENTED_EDGE('',*,*,#2186,.F.);
#3142=ORIENTED_EDGE('',*,*,#2183,.F.);
#3143=ORIENTED_EDGE('',*,*,#2184,.F.);
#3144=ORIENTED_EDGE('',*,*,#2181,.F.);
#3145=ORIENTED_EDGE('',*,*,#2180,.F.);
#3146=ORIENTED_EDGE('',*,*,#2186,.T.);
#3147=ORIENTED_EDGE('',*,*,#2187,.T.);
#3148=ORIENTED_EDGE('',*,*,#2187,.F.);
#3149=ORIENTED_EDGE('',*,*,#2185,.F.);
#3421=ADVANCED_FACE('',(#509),#133,.T.);
#3422=ADVANCED_FACE('',(#510,#223),#134,.T.);
#3423=ADVANCED_FACE('',(#511),#47,.F.);
#3424=ADVANCED_FACE('',(#512),#48,.F.);
#3425=ADVANCED_FACE('',(#513),#293,.F.);
#3434=CLOSED_SHELL('',(#3421));
#3435=CLOSED_SHELL('',(#3422,#3423,#3424,#3425));
#4016=AXIS2_PLACEMENT_3D('',#8368,#5193,#5194);
#4017=AXIS2_PLACEMENT_3D('',#8369,#5195,#5196);
#4018=AXIS2_PLACEMENT_3D('',#8371,#5197,#5198);
#4019=AXIS2_PLACEMENT_3D('',#8372,#5199,#5200);
#4020=AXIS2_PLACEMENT_3D('',#8373,#5201,#5202);
#4021=AXIS2_PLACEMENT_3D('',#8375,#5203,#5204);
#4022=AXIS2_PLACEMENT_3D('',#8376,#5205,#5206);
#4023=AXIS2_PLACEMENT_3D('',#8435,#5207,#5208);
#4024=AXIS2_PLACEMENT_3D('',#9478,#5209,#5210);
#4025=AXIS2_PLACEMENT_3D('',#10519,#5211,#5212);
#4026=AXIS2_PLACEMENT_3D('',#10520,#5213,#5214);
#5193=DIRECTION('axis',(0.,0.,1.));
#5194=DIRECTION('refdir',(1.,0.,0.));
#5195=DIRECTION('center_axis',(0.,-1.,0.));
#5196=DIRECTION('ref_axis',(0.,0.,-1.));
#5197=DIRECTION('center_axis',(-1.,0.,-1.22464679914735E-16));
#5198=DIRECTION('ref_axis',(-1.22464679914735E-16,0.,1.));
#5199=DIRECTION('center_axis',(0.,1.,0.));
#5200=DIRECTION('ref_axis',(0.,0.,-1.));
#5201=DIRECTION('center_axis',(0.,-1.,0.));
#5202=DIRECTION('ref_axis',(0.,0.,-1.));
#5203=DIRECTION('center_axis',(-1.,0.,-1.22464679914735E-16));
#5204=DIRECTION('ref_axis',(-1.22464679914735E-16,0.,1.));
#5205=DIRECTION('center_axis',(0.,1.,0.));
#5206=DIRECTION('ref_axis',(0.,0.,-1.));
#5207=DIRECTION('center_axis',(0.715813339017001,0.0683962349942489,-0.694933967168064));
#5208=DIRECTION('ref_axis',(0.0832680595661294,0.979730076642959,0.182196067952284));
#5209=DIRECTION('center_axis',(0.721009996323288,0.136469090742821,-0.679353201562869));
#5210=DIRECTION('ref_axis',(-0.685769030757116,2.74420183243792E-16,-0.727819233363921));
#5211=DIRECTION('center_axis',(0.721009996323288,0.136469090742821,-0.679353201562869));
#5212=DIRECTION('ref_axis',(-0.685769030757116,2.74420183243792E-16,-0.727819233363921));
#5213=DIRECTION('center_axis',(0.721009996323288,0.136469090742821,-0.679353201562869));
#5214=DIRECTION('ref_axis',(-0.685769030757116,9.43576066543432E-18,-0.727819233363921));
#8368=CARTESIAN_POINT('',(0.,0.,0.));
#8369=CARTESIAN_POINT('Origin',(0.,0.,0.));
#8370=CARTESIAN_POINT('',(-6.58247654541702E-16,-2.14313189850787E-17,5.375));
#8371=CARTESIAN_POINT('Origin',(-6.79678973526781E-16,0.,5.55));
#8372=CARTESIAN_POINT('Origin',(0.,2.14313189850787E-17,0.));
#8373=CARTESIAN_POINT('Origin',(0.,11.,0.));
#8374=CARTESIAN_POINT('',(-3.67484018169097E-16,11.,3.00073472959676));
#8375=CARTESIAN_POINT('Origin',(-3.88915337154176E-16,11.,3.17573472959676));
#8376=CARTESIAN_POINT('Origin',(0.,11.,0.));
#8377=CARTESIAN_POINT('',(-2.3674783363584,10.9996616868026,-2.37117425835928));
#8378=CARTESIAN_POINT('',(-2.36654172903753,11.0369221330747,-2.36654172907039));
#8379=CARTESIAN_POINT('Ctrl Pts',(-2.36654172902905,11.0369221332381,-2.36654172902901));
#8380=CARTESIAN_POINT('Ctrl Pts',(-2.36660261520315,11.0363244725787,-2.36666327705626));
#8381=CARTESIAN_POINT('Ctrl Pts',(-2.36666128562436,11.0357261397191,-2.36678260888203));
#8382=CARTESIAN_POINT('Ctrl Pts',(-2.36723393352068,11.029650121596,-2.36797057219123));
#8383=CARTESIAN_POINT('Ctrl Pts',(-2.36756434090361,11.0241223710425,-2.36885504265911));
#8384=CARTESIAN_POINT('Ctrl Pts',(-2.36786981099157,11.0122851763974,-2.37033490110904));
#8385=CARTESIAN_POINT('Ctrl Pts',(-2.36779322640185,11.0059755411538,-2.37087710768974));
#8386=CARTESIAN_POINT('Ctrl Pts',(-2.36747833635822,10.9996616867988,-2.37117425835944));
#8387=CARTESIAN_POINT('',(-2.45534485149915,10.9282219455009,-1.7516666854678));
#8388=CARTESIAN_POINT('Ctrl Pts',(-2.36654172902905,11.0369221332381,-2.36654172902902));
#8389=CARTESIAN_POINT('Ctrl Pts',(-2.37334411896229,11.0362823302019,-2.35993463713669));
#8390=CARTESIAN_POINT('Ctrl Pts',(-2.38011577585649,11.0356428039708,-2.35329589463348));
#8391=CARTESIAN_POINT('Ctrl Pts',(-2.54314617762233,11.0201812306806,-2.19197276001336));
#8392=CARTESIAN_POINT('Ctrl Pts',(-2.68269334753296,11.0055217449001,-2.0205521909063));
#8393=CARTESIAN_POINT('Ctrl Pts',(-2.93077377794738,10.9744992833803,-1.63885953638735));
#8394=CARTESIAN_POINT('Ctrl Pts',(-3.03643612092201,10.9580589959793,-1.42666947885773));
#8395=CARTESIAN_POINT('Ctrl Pts',(-3.24828372828744,10.9112686417533,-0.832197869920266));
#8396=CARTESIAN_POINT('Ctrl Pts',(-3.28050325458791,10.8850718442332,-0.503072235115654));
#8397=CARTESIAN_POINT('Ctrl Pts',(-3.27116719523908,10.8542407041749,-0.173247696238549));
#8398=CARTESIAN_POINT('Ctrl Pts',(-3.25839405608137,10.8451986333149,-0.0885221583575347));
#8399=CARTESIAN_POINT('Ctrl Pts',(-3.23881660723628,10.8367580084259,-0.0305206064263497));
#8400=CARTESIAN_POINT('Ctrl Pts',(-3.23350366077321,10.8346759734772,-0.0174528173977804));
#8401=CARTESIAN_POINT('Ctrl Pts',(-3.22490854320742,10.8320397599134,-0.00643610865276417));
#8402=CARTESIAN_POINT('Ctrl Pts',(-3.22255570142893,10.8313575488208,-0.00396872044824001));
#8403=CARTESIAN_POINT('Ctrl Pts',(-3.21825792744808,10.8302367058123,-0.00122700918978464));
#8404=CARTESIAN_POINT('Ctrl Pts',(-3.21649608927482,10.8298022464972,-0.000455877488832637));
#8405=CARTESIAN_POINT('Ctrl Pts',(-3.21302387578014,10.8290112656581,0.000142774382210926));
#8406=CARTESIAN_POINT('Ctrl Pts',(-3.21144786498889,10.828675339728,8.85061552719118E-5));
#8407=CARTESIAN_POINT('Ctrl Pts',(-3.20813643512089,10.8280166434058,-0.000687603043136314));
#8408=CARTESIAN_POINT('Ctrl Pts',(-3.2065013980317,10.8277189617055,-0.00145760483001095));
#8409=CARTESIAN_POINT('Ctrl Pts',(-3.20251334962923,10.8270431196483,-0.00403322970158444));
#8410=CARTESIAN_POINT('Ctrl Pts',(-3.20028633028751,10.8267209281034,-0.00623711459830585));
#8411=CARTESIAN_POINT('Ctrl Pts',(-3.19410520074952,10.8259164744266,-0.0135679320571353));
#8412=CARTESIAN_POINT('Ctrl Pts',(-3.19023496381139,10.8255747732312,-0.0203458579147062));
#8413=CARTESIAN_POINT('Ctrl Pts',(-3.1768815605095,10.8247309008079,-0.0479485545610701));
#8414=CARTESIAN_POINT('Ctrl Pts',(-3.16735042929677,10.8249800714079,-0.0783448786336477));
#8415=CARTESIAN_POINT('Ctrl Pts',(-3.11478686213639,10.8290765772632,-0.269802373389443));
#8416=CARTESIAN_POINT('Ctrl Pts',(-3.06060090440076,10.843895246432,-0.566826036283537));
#8417=CARTESIAN_POINT('Ctrl Pts',(-2.86004093617191,10.876114649494,-1.07584184708214));
#8418=CARTESIAN_POINT('Ctrl Pts',(-2.78959762400602,10.8863469276679,-1.22442516795858));
#8419=CARTESIAN_POINT('Ctrl Pts',(-2.66904925825053,10.9023565788694,-1.43719223473247));
#8420=CARTESIAN_POINT('Ctrl Pts',(-2.62779792624269,10.9076260262076,-1.50448086866193));
#8421=CARTESIAN_POINT('Ctrl Pts',(-2.5432634370422,10.917999580532,-1.63214960111092));
#8422=CARTESIAN_POINT('Ctrl Pts',(-2.50029161260727,10.9230894885434,-1.69263839311565));
#8423=CARTESIAN_POINT('Ctrl Pts',(-2.45534485149905,10.9282219455009,-1.75166668546793));
#8424=CARTESIAN_POINT('',(-2.12462539575998,10.9630778666627,-2.12462539640225));
#8425=CARTESIAN_POINT('Ctrl Pts',(-2.45534485149915,10.9282219455009,-1.7516666854678));
#8426=CARTESIAN_POINT('Ctrl Pts',(-2.40908054625928,10.9335048524215,-1.81242530005626));
#8427=CARTESIAN_POINT('Ctrl Pts',(-2.3606379133253,10.9388413422232,-1.87174235306124));
#8428=CARTESIAN_POINT('Ctrl Pts',(-2.31017054130683,10.9442027102673,-1.92935832892452));
#8429=CARTESIAN_POINT('Ctrl Pts',(-2.26186164921788,10.949334773617,-1.98451008042768));
#8430=CARTESIAN_POINT('Ctrl Pts',(-2.21169772289672,10.9544892409942,-2.03810240827354));
#8431=CARTESIAN_POINT('Ctrl Pts',(-2.15984481067586,10.9596213484018,-2.08993852779845));
#8432=CARTESIAN_POINT('Ctrl Pts',(-2.14818952039214,10.960774922985,-2.10159004348713));
#8433=CARTESIAN_POINT('Ctrl Pts',(-2.13644901713658,10.9619273010852,-2.11315298186845));
#8434=CARTESIAN_POINT('Ctrl Pts',(-2.12462539575998,10.9630778666627,-2.12462539640225));
#8435=CARTESIAN_POINT('Origin',(-2.24558440890951,11.0000054639071,-2.24558417873147));
#8436=CARTESIAN_POINT('Ctrl Pts',(-2.36456791311707,11.0001838839337,-2.37391751282759));
#8437=CARTESIAN_POINT('Ctrl Pts',(-2.68439695740737,10.9428309226217,-2.07282384920463));
#8438=CARTESIAN_POINT('Ctrl Pts',(-2.94593475213736,10.885477961311,-1.70638527343931));
#8439=CARTESIAN_POINT('Ctrl Pts',(-3.30964371429254,10.7708333333336,-0.896538039613314));
#8440=CARTESIAN_POINT('Ctrl Pts',(-3.41180604852602,10.7135416666669,-0.453515668913589));
#8441=CARTESIAN_POINT('Ctrl Pts',(-3.4379002366457,10.5989583333331,0.443108774718904));
#8442=CARTESIAN_POINT('Ctrl Pts',(-3.36178304590245,10.5416666666666,0.896358100460257));
#8443=CARTESIAN_POINT('Ctrl Pts',(-3.03905091217473,10.4270833333334,1.74368979436799));
#8444=CARTESIAN_POINT('Ctrl Pts',(-2.79252711081109,10.3697916666664,2.13742396723561));
#8445=CARTESIAN_POINT('Ctrl Pts',(-2.16323413009096,10.2552083333337,2.80361970275416));
#8446=CARTESIAN_POINT('Ctrl Pts',(-1.78068510549046,10.1979166666664,3.07579175088966));
#8447=CARTESIAN_POINT('Ctrl Pts',(-0.935379221363662,10.0833333333336,3.45417305821104));
#8448=CARTESIAN_POINT('Ctrl Pts',(-0.472940081479242,10.0260416666666,3.56019762788479));
#8449=CARTESIAN_POINT('Ctrl Pts',(0.462533187284589,9.91145833333345,3.58629181608734));
#8450=CARTESIAN_POINT('Ctrl Pts',(0.935199282188079,9.85416666666669,3.50631238974053));
#8451=CARTESIAN_POINT('Ctrl Pts',(1.81842261051809,9.73958333333332,3.16871345434639));
#8452=CARTESIAN_POINT('Ctrl Pts',(2.22861752543397,9.68229166666673,2.91119093668731));
#8453=CARTESIAN_POINT('Ctrl Pts',(2.92228352868554,9.56770833333328,2.25442768834444));
#8454=CARTESIAN_POINT('Ctrl Pts',(3.20545429299277,9.51041666666666,1.85541792160244));
#8455=CARTESIAN_POINT('Ctrl Pts',(3.59870240211769,9.39583333333334,0.974220403129539));
#8456=CARTESIAN_POINT('Ctrl Pts',(3.70858920724845,9.3385416666664,0.492364494026195));
#8457=CARTESIAN_POINT('Ctrl Pts',(3.73468339552408,9.22395833333361,-0.481957599831572));
#8458=CARTESIAN_POINT('Ctrl Pts',(3.65084173357628,9.16666666666689,-0.974040463933888));
#8459=CARTESIAN_POINT('Ctrl Pts',(3.29837599652037,9.05208333333312,-1.8931554266502));
#8460=CARTESIAN_POINT('Ctrl Pts',(3.02985476255422,8.99479166666641,-2.31981108364774));
#8461=CARTESIAN_POINT('Ctrl Pts',(2.34562124660724,8.8802083333336,-3.04094735460153));
#8462=CARTESIAN_POINT('Ctrl Pts',(1.93015073770027,8.82291666666647,-3.33511683510577));
#8463=CARTESIAN_POINT('Ctrl Pts',(1.01306158490958,8.70833333333354,-3.74323174601444));
#8464=CARTESIAN_POINT('Ctrl Pts',(0.511788906557484,8.6510416666665,-3.85698078661577));
#8465=CARTESIAN_POINT('Ctrl Pts',(-0.501382012362897,8.53645833333351,-3.88307497495716));
#8466=CARTESIAN_POINT('Ctrl Pts',(-1.01288164569554,8.47916666666683,-3.79537107740945));
#8467=CARTESIAN_POINT('Ctrl Pts',(-1.96788824276646,8.36458333333318,-3.42803853869692));
#8468=CARTESIAN_POINT('Ctrl Pts',(-2.41100464187403,8.30729166666683,-3.14851858841386));
#8469=CARTESIAN_POINT('Ctrl Pts',(-3.159611180505,8.1927083333332,-2.43681480487731));
#8470=CARTESIAN_POINT('Ctrl Pts',(-3.46477937722837,8.13541666666656,-2.00488355378617));
#8471=CARTESIAN_POINT('Ctrl Pts',(-3.8877610899016,8.02083333333345,-1.05190276670153));
#8472=CARTESIAN_POINT('Ctrl Pts',(-4.00537236598643,7.96354166666637,-0.531213319073915));
#8473=CARTESIAN_POINT('Ctrl Pts',(-4.03146655438691,7.84895833333365,0.520806424879362));
#8474=CARTESIAN_POINT('Ctrl Pts',(-3.93990042124014,7.79166666666665,1.05172282747159));
#8475=CARTESIAN_POINT('Ctrl Pts',(-3.55770108087595,7.67708333333337,2.04262105886835));
#8476=CARTESIAN_POINT('Ctrl Pts',(-3.26718241426475,7.61979166666659,2.50219820011361));
#8477=CARTESIAN_POINT('Ctrl Pts',(-2.52800836315612,7.50520833333343,3.27827500639517));
#8478=CARTESIAN_POINT('Ctrl Pts',(-2.07961636986072,7.44791666666668,3.59444191935829));
#8479=CARTESIAN_POINT('Ctrl Pts',(-1.09074394850484,7.33333333333333,4.03229043378143));
#8480=CARTESIAN_POINT('Ctrl Pts',(-0.550637731576509,7.27604166666629,4.15376394536062));
#8481=CARTESIAN_POINT('Ctrl Pts',(0.540230837381994,7.16145833333372,4.17985813381312));
#8482=CARTESIAN_POINT('Ctrl Pts',(1.09056400926098,7.10416666666678,4.08442976506864));
#8483=CARTESIAN_POINT('Ctrl Pts',(2.11735387495688,6.98958333333323,3.68736362305719));
#8484=CARTESIAN_POINT('Ctrl Pts',(2.59339175836345,6.93229166666724,3.38584624010982));
#8485=CARTESIAN_POINT('Ctrl Pts',(3.3969388322751,6.81770833333277,2.61920192144075));
#8486=CARTESIAN_POINT('Ctrl Pts',(3.72410446149635,6.76041666666712,2.15434918592434));
#8487=CARTESIAN_POINT('Ctrl Pts',(4.17681977765313,6.64583333333289,1.12958513031907));
#8488=CARTESIAN_POINT('Ctrl Pts',(4.30215552473732,6.58854166666688,0.570062144068889));
#8489=CARTESIAN_POINT('Ctrl Pts',(4.32824971323683,6.47395833333313,-0.559655249874413));
#8490=CARTESIAN_POINT('Ctrl Pts',(4.22895910889563,6.41666666666645,-1.12940519106012));
#8491=CARTESIAN_POINT('Ctrl Pts',(3.81702616523991,6.30208333333356,-2.19208669103568));
#8492=CARTESIAN_POINT('Ctrl Pts',(3.50451006594675,6.24479166666656,-2.68458531662391));
#8493=CARTESIAN_POINT('Ctrl Pts',(2.71039547973352,6.13020833333345,-3.51560265814439));
#8494=CARTESIAN_POINT('Ctrl Pts',(2.22908200197935,6.07291666666717,-3.85376700363998));
#8495=CARTESIAN_POINT('Ctrl Pts',(1.16842631214193,5.95833333333284,-4.32134912151925));
#8496=CARTESIAN_POINT('Ctrl Pts',(0.589486556547344,5.90104166666655,-4.45054710411593));
#8497=CARTESIAN_POINT('Ctrl Pts',(-0.579079662352908,5.78645833333346,-4.47664129265863));
#8498=CARTESIAN_POINT('Ctrl Pts',(-1.16824637287424,5.72916666666705,-4.37348845271886));
#8499=CARTESIAN_POINT('Ctrl Pts',(-2.26681950709949,5.61458333333296,-3.94668870742641));
#8500=CARTESIAN_POINT('Ctrl Pts',(-2.77577887489086,5.55729166666709,-3.62317389178086));
#8501=CARTESIAN_POINT('Ctrl Pts',(-3.6342664840072,5.44270833333292,-2.80158903802911));
#8502=CARTESIAN_POINT('Ctrl Pts',(-3.98342954578962,5.38541666666669,-2.30381481802579));
#8503=CARTESIAN_POINT('Ctrl Pts',(-4.46587846537937,5.27083333333332,-1.20726749397333));
#8504=CARTESIAN_POINT('Ctrl Pts',(-4.59893868349712,5.21354166666665,-0.608910969019916));
#8505=CARTESIAN_POINT('Ctrl Pts',(-4.62503287207784,5.09895833333335,0.598504074825539));
#8506=CARTESIAN_POINT('Ctrl Pts',(-4.51801779654147,5.04166666666663,1.20708755469526));
#8507=CARTESIAN_POINT('Ctrl Pts',(-4.07635124961353,4.92708333333338,2.34155232315641));
#8508=CARTESIAN_POINT('Ctrl Pts',(-3.74183771760646,4.86979166666659,2.86697243316876));
#8509=CARTESIAN_POINT('Ctrl Pts',(-2.89278259633321,4.75520833333342,3.75293030985906));
#8510=CARTESIAN_POINT('Ctrl Pts',(-2.37854763406351,4.69791666666658,4.1130920879442));
#8511=CARTESIAN_POINT('Ctrl Pts',(-1.24610867581347,4.58333333333343,4.61040780923455));
#8512=CARTESIAN_POINT('Ctrl Pts',(-0.628335381481812,4.52604166666658,4.74733026287932));
#8513=CARTESIAN_POINT('Ctrl Pts',(0.617928487287482,4.41145833333343,4.77342445149605));
#8514=CARTESIAN_POINT('Ctrl Pts',(1.24592873652376,4.35416666666679,4.66254714036264));
#8515=CARTESIAN_POINT('Ctrl Pts',(2.41628513920584,4.23958333333322,4.20601379180208));
#8516=CARTESIAN_POINT('Ctrl Pts',(2.95816599145146,4.18229166666676,3.86050154342994));
#8517=CARTESIAN_POINT('Ctrl Pts',(3.87159413570613,4.06770833333325,2.98397615463943));
#8518=CARTESIAN_POINT('Ctrl Pts',(4.24275463010319,4.01041666666671,2.45328045009706));
#8519=CARTESIAN_POINT('Ctrl Pts',(4.75493715308532,3.8958333333333,1.28494985765777));
#8520=CARTESIAN_POINT('Ctrl Pts',(4.89572184226387,3.83854166666642,0.647759793932574));
#8521=CARTESIAN_POINT('Ctrl Pts',(4.9218160309119,3.72395833333359,-0.637352899738291));
#8522=CARTESIAN_POINT('Ctrl Pts',(4.80707648417982,3.66666666666662,-1.28476991836542));
#8523=CARTESIAN_POINT('Ctrl Pts',(4.33567633399462,3.55208333333339,-2.49101795524214));
#8524=CARTESIAN_POINT('Ctrl Pts',(3.97916536924807,3.49479166666671,-3.04935954974168));
#8525=CARTESIAN_POINT('Ctrl Pts',(3.075169712951,3.38020833333329,-3.99025796154567));
#8526=CARTESIAN_POINT('Ctrl Pts',(2.52801326612096,3.3229166666668,-4.37241717226731));
#8527=CARTESIAN_POINT('Ctrl Pts',(1.3237910395117,3.20833333333321,-4.89946649693097));
#8528=CARTESIAN_POINT('Ctrl Pts',(0.667184206381905,3.15104166666636,-5.04411342164931));
#8529=CARTESIAN_POINT('Ctrl Pts',(-0.656777312187654,3.03645833333365,-5.07020761032686));
#8530=CARTESIAN_POINT('Ctrl Pts',(-1.32361110020785,2.97916666666654,-4.95160582799841));
#8531=CARTESIAN_POINT('Ctrl Pts',(-2.56575077127763,2.86458333333347,-4.46533887618575));
#8532=CARTESIAN_POINT('Ctrl Pts',(-3.1405531080382,2.80729166666695,-4.09782919506089));
#8533=CARTESIAN_POINT('Ctrl Pts',(-4.10892178737893,2.69270833333305,-3.16636327126786));
#8534=CARTESIAN_POINT('Ctrl Pts',(-4.50207971443576,2.63541666666658,-2.60274608213879));
#8535=CARTESIAN_POINT('Ctrl Pts',(-5.04399584077227,2.52083333333343,-1.36263222137173));
#8536=CARTESIAN_POINT('Ctrl Pts',(-5.1925050010359,2.4635416666663,-0.686608618821642));
#8537=CARTESIAN_POINT('Ctrl Pts',(-5.21859918974068,2.34895833333371,0.67620172462746));
#8538=CARTESIAN_POINT('Ctrl Pts',(-5.09613517181383,2.29166666666676,1.36245228206106));
#8539=CARTESIAN_POINT('Ctrl Pts',(-4.59500141838005,2.17708333333325,2.64048358730238));
#8540=CARTESIAN_POINT('Ctrl Pts',(-4.21649302087059,2.11979166666664,3.23174666634004));
#8541=CARTESIAN_POINT('Ctrl Pts',(-3.25755682958786,2.00520833333337,4.22758561320685));
#8542=CARTESIAN_POINT('Ctrl Pts',(-2.67747889815098,1.94791666666658,4.63174225660692));
#8543=CARTESIAN_POINT('Ctrl Pts',(-1.40147340323737,1.83333333333343,5.18852518461089));
#8544=CARTESIAN_POINT('Ctrl Pts',(-0.706033031254986,1.77604166666627,5.34089658042353));
#8545=CARTESIAN_POINT('Ctrl Pts',(0.695626137060878,1.66145833333374,5.36699076915345));
#8546=CARTESIAN_POINT('Ctrl Pts',(1.40129346391331,1.60416666666663,5.24066451563091));
#8547=CARTESIAN_POINT('Ctrl Pts',(2.71521640332806,1.48958333333338,4.7246639605727));
#8548=CARTESIAN_POINT('Ctrl Pts',(3.32294022464786,1.43229166666683,4.33515684667557));
#8549=CARTESIAN_POINT('Ctrl Pts',(4.34624943902881,1.31770833333318,3.34875038791256));
#8550=CARTESIAN_POINT('Ctrl Pts',(4.76140479878007,1.26041666666641,2.75221171416214));
#8551=CARTESIAN_POINT('Ctrl Pts',(5.3330545284475,1.1458333333336,1.44031458510402));
#8552=CARTESIAN_POINT('Ctrl Pts',(5.48928815981245,1.08854166666688,0.72545744367903));
#8553=CARTESIAN_POINT('Ctrl Pts',(5.51538234856494,0.973958333333134,-0.715050549484959));
#8554=CARTESIAN_POINT('Ctrl Pts',(5.38519385944284,0.916666666666909,-1.44013464577813));
#8555=CARTESIAN_POINT('Ctrl Pts',(4.85432650277048,0.8020833333331,-2.7899492193412));
#8556=CARTESIAN_POINT('Ctrl Pts',(4.4538206724838,0.744791666666392,-3.4141337829535));
#8557=CARTESIAN_POINT('Ctrl Pts',(3.43994394623404,0.630208333333619,-4.46491326485293));
#8558=CARTESIAN_POINT('Ctrl Pts',(2.82694453016243,0.572916666666411,-4.89106734095877));
#8559=CARTESIAN_POINT('Ctrl Pts',(1.47915576698159,0.4583333333336,-5.47758387227856));
#8560=CARTESIAN_POINT('Ctrl Pts',(0.744881856102772,0.401041666666677,-5.63767973920226));
#8561=CARTESIAN_POINT('Ctrl Pts',(-0.73447496190878,0.286458333333334,-5.66377392797554));
#8562=CARTESIAN_POINT('Ctrl Pts',(-1.4789758276525,0.229166666666838,-5.52972320325324));
#8563=CARTESIAN_POINT('Ctrl Pts',(-2.86468203534475,0.114583333333173,-4.9839890449698));
#8564=CARTESIAN_POINT('Ctrl Pts',(-3.50532733285514,0.0572916666665569,
-4.5724845058884));
#8565=CARTESIAN_POINT('Ctrl Pts',(-4.04445221596811,5.20417042793042E-15,
-4.05181100142375));
#8566=CARTESIAN_POINT('Ctrl Pts',(-2.39934536183762,11.346909399206,-2.34117692464435));
#8567=CARTESIAN_POINT('Ctrl Pts',(-2.71488410852275,11.2895564378939,-2.03552600632456));
#8568=CARTESIAN_POINT('Ctrl Pts',(-2.9712261341221,11.2322034765833,-1.66538602697384));
#8569=CARTESIAN_POINT('Ctrl Pts',(-3.32352361490692,11.1175588486058,-0.850409340498224));
#8570=CARTESIAN_POINT('Ctrl Pts',(-3.4194758201212,11.0602671819391,-0.405958512493029));
#8571=CARTESIAN_POINT('Ctrl Pts',(-3.43307090382695,10.9456838486053,0.491037743700738));
#8572=CARTESIAN_POINT('Ctrl Pts',(-3.35066965504748,10.8883921819389,0.943230278421825));
#8573=CARTESIAN_POINT('Ctrl Pts',(-3.01624756806638,10.7738088486056,1.78612228216488));
#8574=CARTESIAN_POINT('Ctrl Pts',(-2.76432247051982,10.7165171819386,2.17647530254211));
#8575=CARTESIAN_POINT('Ctrl Pts',(-2.12592837712132,10.6019338486059,2.83409574774927));
#8576=CARTESIAN_POINT('Ctrl Pts',(-1.7396831165707,10.5446421819387,3.10107703174287));
#8577=CARTESIAN_POINT('Ctrl Pts',(-0.889250522245734,10.4300588486058,3.46805295881896));
#8578=CARTESIAN_POINT('Ctrl Pts',(-0.425382925058827,10.3727671819388,3.56786739948684));
#8579=CARTESIAN_POINT('Ctrl Pts',(0.510462156266568,10.2581838486057,3.58146248326171));
#8580=CARTESIAN_POINT('Ctrl Pts',(0.982071460151994,10.2008921819389,3.49519899889172));
#8581=CARTESIAN_POINT('Ctrl Pts',(1.86085509831263,10.0863088486056,3.14591011023186));
#8582=CARTESIAN_POINT('Ctrl Pts',(2.26766886074488,10.029017181939,2.88298629640079));
#8583=CARTESIAN_POINT('Ctrl Pts',(2.95275957367625,9.91443384860552,2.21712193537007));
#8584=CARTESIAN_POINT('Ctrl Pts',(3.2307395738517,9.8571421819389,1.81441593268519));
#8585=CARTESIAN_POINT('Ctrl Pts',(3.61258230271989,9.74255884860558,0.9280917040091));
#8586=CARTESIAN_POINT('Ctrl Pts',(3.71625897885657,9.68526718193864,0.444807337606009));
#8587=CARTESIAN_POINT('Ctrl Pts',(3.72985406269238,9.57068384860585,-0.52988656881378));
#8588=CARTESIAN_POINT('Ctrl Pts',(3.63972834273301,9.51339218193913,-1.02091264189992));
#8589=CARTESIAN_POINT('Ctrl Pts',(3.2755726524003,9.39880884860535,-1.93558791444263));
#8590=CARTESIAN_POINT('Ctrl Pts',(3.00165012227183,9.34151718193865,-2.35886241896257));
#8591=CARTESIAN_POINT('Ctrl Pts',(2.30831549362873,9.22693384860584,-3.07142339958832));
#8592=CARTESIAN_POINT('Ctrl Pts',(1.88914874878537,9.1696421819387,-3.3604021159697));
#8593=CARTESIAN_POINT('Ctrl Pts',(0.966932885786784,9.05505884860578,-3.75711164661164));
#8594=CARTESIAN_POINT('Ctrl Pts',(0.46423175013744,8.99776718193874,-3.86465055822945));
#8595=CARTESIAN_POINT('Ctrl Pts',(-0.549310981345248,8.88318384860575,-3.87824564211992));
#8596=CARTESIAN_POINT('Ctrl Pts',(-1.05975382366345,8.82589218193907,-3.78425768657106));
#8597=CARTESIAN_POINT('Ctrl Pts',(-2.01032073055702,8.71130884860541,-3.40523519457197));
#8598=CARTESIAN_POINT('Ctrl Pts',(-2.45005597719243,8.65401718193906,-3.12031394813519));
#8599=CARTESIAN_POINT('Ctrl Pts',(-3.19008722548821,8.53943384860543,-2.39950905189507));
#8600=CARTESIAN_POINT('Ctrl Pts',(-3.49006465809683,8.4821421819388,-1.96388156487328));
#8601=CARTESIAN_POINT('Ctrl Pts',(-3.90164099049427,8.36755884860569,-1.00577406757673));
#8602=CARTESIAN_POINT('Ctrl Pts',(-4.01304213760465,8.3102671819386,-0.483656162654029));
#8603=CARTESIAN_POINT('Ctrl Pts',(-4.02663722154512,8.19568384860588,0.568735393861871));
#8604=CARTESIAN_POINT('Ctrl Pts',(-3.92878703040616,8.13839218193865,1.09859500544122));
#8605=CARTESIAN_POINT('Ctrl Pts',(-3.5348977367466,8.02380884860583,2.08505354665718));
#8606=CARTESIAN_POINT('Ctrl Pts',(-3.23897777398945,7.96651718193906,2.54124953543508));
#8607=CARTESIAN_POINT('Ctrl Pts',(-2.49070261017052,7.85193384860543,3.30875105137532));
#8608=CARTESIAN_POINT('Ctrl Pts',(-2.03861438094966,7.79464218193892,3.61972720023077));
#8609=CARTESIAN_POINT('Ctrl Pts',(-1.0446152493782,7.68005884860556,4.04617033437007));
#8610=CARTESIAN_POINT('Ctrl Pts',(-0.503080575156725,7.62276718193853,4.16143371698328));
#8611=CARTESIAN_POINT('Ctrl Pts',(0.588159806364604,7.50818384860596,4.17502880096689));
#8612=CARTESIAN_POINT('Ctrl Pts',(1.13743618723204,7.45089218193902,4.07331637423875));
#8613=CARTESIAN_POINT('Ctrl Pts',(2.15978636274428,7.33630884860546,3.66456027892374));
#8614=CARTESIAN_POINT('Ctrl Pts',(2.63244309368768,7.27901718193947,3.35764159983753));
#8615=CARTESIAN_POINT('Ctrl Pts',(3.42741487725249,7.16443384860501,2.58189616845213));
#8616=CARTESIAN_POINT('Ctrl Pts',(3.74938974237272,7.10714218193936,2.11334719701498));
#8617=CARTESIAN_POINT('Ctrl Pts',(4.19069967823789,6.99255884860513,1.08345643119075));
#8618=CARTESIAN_POINT('Ctrl Pts',(4.30982529636403,6.93526718193912,0.522504987649244));
#8619=CARTESIAN_POINT('Ctrl Pts',(4.32342038038655,6.82068384860537,-0.607584218857162));
#8620=CARTESIAN_POINT('Ctrl Pts',(4.21784571806929,6.76339218193869,-1.17627736903264));
#8621=CARTESIAN_POINT('Ctrl Pts',(3.79422282110293,6.6488088486058,-2.23451917882162));
#8622=CARTESIAN_POINT('Ctrl Pts',(3.47630542567715,6.5915171819388,-2.72363665195073));
#8623=CARTESIAN_POINT('Ctrl Pts',(2.67308972674222,6.47693384860569,-3.54607870311919));
#8624=CARTESIAN_POINT('Ctrl Pts',(2.18808001307138,6.41964218193941,-3.87905228451955));
#8625=CARTESIAN_POINT('Ctrl Pts',(1.1222976130122,6.30505884860508,-4.33522902210081));
#8626=CARTESIAN_POINT('Ctrl Pts',(0.541929400127819,6.24776718193879,-4.45821687574607));
#8627=CARTESIAN_POINT('Ctrl Pts',(-0.627008631335778,6.1331838486057,-4.47181195980492));
#8628=CARTESIAN_POINT('Ctrl Pts',(-1.21511855084784,6.07589218193929,-4.3623750618956));
#8629=CARTESIAN_POINT('Ctrl Pts',(-2.30925199488436,5.9613088486052,-3.92388536328634));
#8630=CARTESIAN_POINT('Ctrl Pts',(-2.81483021022013,5.90401718193932,-3.59496925151373));
#8631=CARTESIAN_POINT('Ctrl Pts',(-3.66474252897955,5.78943384860516,-2.76428328503534));
#8632=CARTESIAN_POINT('Ctrl Pts',(-4.0087148266721,5.73214218193892,-2.26281282911923));
#8633=CARTESIAN_POINT('Ctrl Pts',(-4.47975836595802,5.61755884860556,-1.1611387948422));
#8634=CARTESIAN_POINT('Ctrl Pts',(-4.60660845513052,5.56026718193889,-0.561353812600464));
#8635=CARTESIAN_POINT('Ctrl Pts',(-4.62020353922087,5.44568384860559,0.646433043808482));
#8636=CARTESIAN_POINT('Ctrl Pts',(-4.50690440572112,5.38839218193887,1.25395973267003));
#8637=CARTESIAN_POINT('Ctrl Pts',(-4.05354790547054,5.27380884860562,2.38398481094011));
#8638=CARTESIAN_POINT('Ctrl Pts',(-3.71363307734148,5.21651718193883,2.90602376850005));
#8639=CARTESIAN_POINT('Ctrl Pts',(-2.85547684333729,5.10193384860566,3.78340635482939));
#8640=CARTESIAN_POINT('Ctrl Pts',(-2.33754564515818,5.04464218193881,4.13837736882935));
#8641=CARTESIAN_POINT('Ctrl Pts',(-1.1999799766811,4.93005884860567,4.62428770981052));
#8642=CARTESIAN_POINT('Ctrl Pts',(-0.580778225062417,4.87276718193882,4.75500003451575));
#8643=CARTESIAN_POINT('Ctrl Pts',(0.665857456270481,4.75818384860567,4.76859511863605));
#8644=CARTESIAN_POINT('Ctrl Pts',(1.2928009144995,4.70089218193903,4.65143374954513));
#8645=CARTESIAN_POINT('Ctrl Pts',(2.45871762698856,4.58630884860546,4.18321044765625));
#8646=CARTESIAN_POINT('Ctrl Pts',(2.99721732678471,4.529017181939,3.83229690316695));
#8647=CARTESIAN_POINT('Ctrl Pts',(3.9020701806745,4.41443384860549,2.94667040164152));
#8648=CARTESIAN_POINT('Ctrl Pts',(4.2680399109909,4.35714218193895,2.41227846119283));
#8649=CARTESIAN_POINT('Ctrl Pts',(4.76881705365873,4.24255884860554,1.2388211585243));
#8650=CARTESIAN_POINT('Ctrl Pts',(4.90339161390277,4.18526718193866,0.600202637513305));
#8651=CARTESIAN_POINT('Ctrl Pts',(4.91698669804943,4.07068384860583,-0.685281868721417));
#8652=CARTESIAN_POINT('Ctrl Pts',(4.79596309336461,4.01339218193886,-1.33164209634213));
#8653=CARTESIAN_POINT('Ctrl Pts',(4.31287298984649,3.89880884860562,-2.53345044302389));
#8654=CARTESIAN_POINT('Ctrl Pts',(3.95096072898711,3.84151718193895,-3.08841088507667));
#8655=CARTESIAN_POINT('Ctrl Pts',(3.03786395995105,3.72693384860553,-4.02073400651229));
#8656=CARTESIAN_POINT('Ctrl Pts',(2.48701127721779,3.66964218193904,-4.39770245315732));
#8657=CARTESIAN_POINT('Ctrl Pts',(1.27766234037718,3.55505884860545,-4.91334639750207));
#8658=CARTESIAN_POINT('Ctrl Pts',(0.619627049962736,3.4977671819386,-5.05178319329073));
#8659=CARTESIAN_POINT('Ctrl Pts',(-0.704706281170879,3.38318384860588,-5.06537827746187));
#8660=CARTESIAN_POINT('Ctrl Pts',(-1.37048327818541,3.32589218193878,-4.94049243718524));
#8661=CARTESIAN_POINT('Ctrl Pts',(-2.60818325905853,3.21130884860571,-4.44253553203559));
#8662=CARTESIAN_POINT('Ctrl Pts',(-3.17960444337468,3.15401718193919,-4.06962455480154));
#8663=CARTESIAN_POINT('Ctrl Pts',(-4.13939783234407,3.03943384860528,-3.1290575182663));
#8664=CARTESIAN_POINT('Ctrl Pts',(-4.52736499532796,2.98214218193882,-2.5617440932366));
#8665=CARTESIAN_POINT('Ctrl Pts',(-5.05787574134119,2.86755884860567,-1.31650352223623));
#8666=CARTESIAN_POINT('Ctrl Pts',(-5.20017477267972,2.81026718193854,-0.639051462402516));
#8667=CARTESIAN_POINT('Ctrl Pts',(-5.21376985687329,2.69568384860595,0.724130693610728));
#8668=CARTESIAN_POINT('Ctrl Pts',(-5.08502178100269,2.638392181939,1.40932446003936));
#8669=CARTESIAN_POINT('Ctrl Pts',(-4.57219807422785,2.52380884860549,2.68291607508254));
#8670=CARTESIAN_POINT('Ctrl Pts',(-4.18828838061282,2.46651718193888,3.27079800167798));
#8671=CARTESIAN_POINT('Ctrl Pts',(-3.22025107658473,2.3519338486056,4.25806165817053));
#8672=CARTESIAN_POINT('Ctrl Pts',(-2.63647690924959,2.29464218193882,4.65702753750094));
#8673=CARTESIAN_POINT('Ctrl Pts',(-1.35534470410106,2.18005884860566,5.20240508517798));
#8674=CARTESIAN_POINT('Ctrl Pts',(-0.658475874835927,2.12276718193851,5.34856635206931));
#8675=CARTESIAN_POINT('Ctrl Pts',(0.743555106044213,2.00818384860598,5.3621614362841));
#8676=CARTESIAN_POINT('Ctrl Pts',(1.44816564189249,1.95089218193886,5.22955112482197));
#8677=CARTESIAN_POINT('Ctrl Pts',(2.75764889110733,1.83630884860562,4.70186061641829));
#8678=CARTESIAN_POINT('Ctrl Pts',(3.36199155998716,1.77901718193906,4.30695220641913));
#8679=CARTESIAN_POINT('Ctrl Pts',(4.37672548399112,1.66443384860542,3.3114446349081));
#8680=CARTESIAN_POINT('Ctrl Pts',(4.78669007967579,1.60714218193865,2.71120972526174));
#8681=CARTESIAN_POINT('Ctrl Pts',(5.3469344290129,1.49255884860583,1.39418588596674));
#8682=CARTESIAN_POINT('Ctrl Pts',(5.49695793145999,1.43526718193912,0.677900287260056));
#8683=CARTESIAN_POINT('Ctrl Pts',(5.51055301569383,1.32068384860537,-0.76297951846838));
#8684=CARTESIAN_POINT('Ctrl Pts',(5.37408046863567,1.26339218193915,-1.4870068237579));
#8685=CARTESIAN_POINT('Ctrl Pts',(4.83152315861431,1.14880884860534,-2.83238170711989));
#8686=CARTESIAN_POINT('Ctrl Pts',(4.42561603222875,1.09151718193863,-3.45318511829405));
#8687=CARTESIAN_POINT('Ctrl Pts',(3.40263819322818,0.976933848605856,-4.49538930981399));
#8688=CARTESIAN_POINT('Ctrl Pts',(2.78594254126256,0.919642181938648,-4.91635262185619));
#8689=CARTESIAN_POINT('Ctrl Pts',(1.43302706784377,0.805058848605838,-5.49146377284226));
#8690=CARTESIAN_POINT('Ctrl Pts',(0.697324699683797,0.747767181938915,-5.64534951085169));
#8691=CARTESIAN_POINT('Ctrl Pts',(-0.782403930892199,0.633183848605571,
-5.65894459510253));
#8692=CARTESIAN_POINT('Ctrl Pts',(-1.5258480056327,0.575892181939075,-5.51860981244762));
#8693=CARTESIAN_POINT('Ctrl Pts',(-2.90711452312302,0.46130884860541,-4.96118570081208));
#8694=CARTESIAN_POINT('Ctrl Pts',(-3.54437866826175,0.404017181938794,-4.5442798657039));
#8695=CARTESIAN_POINT('Ctrl Pts',(-4.07921590611891,0.346725515272242,-4.0190558047933));
#8696=CARTESIAN_POINT('Ctrl Pts',(-2.15943324690355,11.346909399206,-2.08633937475486));
#8697=CARTESIAN_POINT('Ctrl Pts',(-2.44157795049855,11.2895564378939,-1.81212632695763));
#8698=CARTESIAN_POINT('Ctrl Pts',(-2.67079732462106,11.2322034765833,-1.48005921159716));
#8699=CARTESIAN_POINT('Ctrl Pts',(-2.98550788648136,11.1175588486058,-0.748702056168519));
#8700=CARTESIAN_POINT('Ctrl Pts',(-3.07099283278885,11.0602671819391,-0.349756983242139));
#8701=CARTESIAN_POINT('Ctrl Pts',(-3.0818633980033,10.9456838486053,0.455650002839366));
#8702=CARTESIAN_POINT('Ctrl Pts',(-3.00720596150024,10.8883921819389,0.861795055291616));
#8703=CARTESIAN_POINT('Ctrl Pts',(-2.70531644391264,10.7738088486056,1.61902697886803));
#8704=CARTESIAN_POINT('Ctrl Pts',(-2.47816730458498,10.7165171819386,1.96980110153648));
#8705=CARTESIAN_POINT('Ctrl Pts',(-1.90261007970139,10.6019338486059,2.56073162722495));
#8706=CARTESIAN_POINT('Ctrl Pts',(-1.55440100825198,10.5446421819387,2.80062812645173));
#8707=CARTESIAN_POINT('Ctrl Pts',(-0.787543237963199,10.4300588486058,3.13003723037197));
#8708=CARTESIAN_POINT('Ctrl Pts',(-0.369181395757753,10.3727671819388,3.21938441215601));
#8709=CARTESIAN_POINT('Ctrl Pts',(0.475074415355009,10.2581838486057,3.23025497743655));
#8710=CARTESIAN_POINT('Ctrl Pts',(0.900636237067393,10.2008921819389,3.15173530532716));
#8711=CARTESIAN_POINT('Ctrl Pts',(1.69375979497017,10.0863088486056,2.83497898609545));
#8712=CARTESIAN_POINT('Ctrl Pts',(2.0609946597737,10.029017181939,2.59683113043342));
#8713=CARTESIAN_POINT('Ctrl Pts',(2.67939545311748,9.91443384860552,1.99380363798266));
#8714=CARTESIAN_POINT('Ctrl Pts',(2.93029066857928,9.8571421819389,1.62913382432459));
#8715=CARTESIAN_POINT('Ctrl Pts',(3.27456657425417,9.74255884860558,0.826384419768452));
#8716=CARTESIAN_POINT('Ctrl Pts',(3.36777599152708,9.68526718193864,0.388605808260406));
#8717=CARTESIAN_POINT('Ctrl Pts',(3.37864655686589,9.57068384860585,-0.49449882785769));
#8718=CARTESIAN_POINT('Ctrl Pts',(3.29626464915295,9.51339218193913,-0.939477418855915));
#8719=CARTESIAN_POINT('Ctrl Pts',(2.96464152827939,9.39880884860535,-1.76849261105957));
#8720=CARTESIAN_POINT('Ctrl Pts',(2.71549495627589,9.34151718193865,-2.15218821802195));
#8721=CARTESIAN_POINT('Ctrl Pts',(2.0849971962699,9.22693384860584,-2.79805927899898));
#8722=CARTESIAN_POINT('Ctrl Pts',(1.70386664038741,9.1696421819387,-3.05995321071421));
#8723=CARTESIAN_POINT('Ctrl Pts',(0.865225601583496,9.05505884860578,-3.419095918129));
#8724=CARTESIAN_POINT('Ctrl Pts',(0.408030220752219,8.99776718193874,-3.51616757090102));
#8725=CARTESIAN_POINT('Ctrl Pts',(-0.513923240349536,8.88318384860575,-3.52703813629236));
#8726=CARTESIAN_POINT('Ctrl Pts',(-0.978318600655415,8.82589218193907,-3.44079399297743));
#8727=CARTESIAN_POINT('Ctrl Pts',(-1.84322542713799,8.71130884860541,-3.09430407046464));
#8728=CARTESIAN_POINT('Ctrl Pts',(-2.24338177627906,8.65401718193906,-2.8341587821133));
#8729=CARTESIAN_POINT('Ctrl Pts',(-2.91672310487163,8.53943384860543,-2.1761907545622));
#8730=CARTESIAN_POINT('Ctrl Pts',(-3.18961575285625,8.4821421819388,-1.77859945644224));
#8731=CARTESIAN_POINT('Ctrl Pts',(-3.56362526199671,8.36755884860569,-0.904066783406526));
#8732=CARTESIAN_POINT('Ctrl Pts',(-3.66455915027763,8.3102671819386,-0.427454633233268));
#8733=CARTESIAN_POINT('Ctrl Pts',(-3.67542971571615,8.19568384860588,0.533347652830617));
#8734=CARTESIAN_POINT('Ctrl Pts',(-3.58532333680026,8.13839218193865,1.01715978246527));
#8735=CARTESIAN_POINT('Ctrl Pts',(-3.22396661265153,8.02380884860583,1.91795824320607));
#8736=CARTESIAN_POINT('Ctrl Pts',(-2.95282260794454,7.96651718193906,2.33457533454633));
#8737=CARTESIAN_POINT('Ctrl Pts',(-2.26738431286067,7.85193384860543,3.03538693073411));
#8738=CARTESIAN_POINT('Ctrl Pts',(-1.85333227248862,7.79464218193892,3.31927829500387));
#8739=CARTESIAN_POINT('Ctrl Pts',(-0.942907965238003,7.68005884860556,3.70815460585884));
#8740=CARTESIAN_POINT('Ctrl Pts',(-0.446879045704217,7.62276718193853,3.81295072965703));
#8741=CARTESIAN_POINT('Ctrl Pts',(0.552772065301601,7.50818384860596,3.82382129513715));
#8742=CARTESIAN_POINT('Ctrl Pts',(1.05600096428514,7.45089218193902,3.7298526806217));
#8743=CARTESIAN_POINT('Ctrl Pts',(1.99269105926411,7.33630884860546,3.35362915483982));
#8744=CARTESIAN_POINT('Ctrl Pts',(2.42576889282071,7.27901718193947,3.07148643377194));
#8745=CARTESIAN_POINT('Ctrl Pts',(3.15405075658949,7.16443384860501,2.35857787116297));
#8746=CARTESIAN_POINT('Ctrl Pts',(3.4489408371573,7.10714218193936,1.92806508852736));
#8747=CARTESIAN_POINT('Ctrl Pts',(3.85268394971518,6.99255884860513,0.981749147077123));
#8748=CARTESIAN_POINT('Ctrl Pts',(3.96134230903857,6.93526718193912,0.466303458167944));
#8749=CARTESIAN_POINT('Ctrl Pts',(3.97221287455602,6.82068384860537,-0.572196477765365));
#8750=CARTESIAN_POINT('Ctrl Pts',(3.87438202444231,6.76339218193869,-1.09484214611198));
#8751=CARTESIAN_POINT('Ctrl Pts',(3.48329169702894,6.6488088486058,-2.06742387531521));
#8752=CARTESIAN_POINT('Ctrl Pts',(3.19015025959274,6.5915171819388,-2.51696245110363));
#8753=CARTESIAN_POINT('Ctrl Pts',(2.44977142947187,6.47693384860569,-3.27271458243633));
#8754=CARTESIAN_POINT('Ctrl Pts',(2.00279790455941,6.41964218193941,-3.57860337931556));
#8755=CARTESIAN_POINT('Ctrl Pts',(1.02059032892293,6.30505884860508,-3.99721329356667));
#8756=CARTESIAN_POINT('Ctrl Pts',(0.485727870620802,6.24776718193879,-4.10973388842147));
#8757=CARTESIAN_POINT('Ctrl Pts',(-0.591620890218261,6.1331838486057,-4.12060445397352));
#8758=CARTESIAN_POINT('Ctrl Pts',(-1.13368332795069,6.07589218193929,-4.01891136825983));
#8759=CARTESIAN_POINT('Ctrl Pts',(-2.14215669135443,5.9613088486052,-3.61295423922114));
#8760=CARTESIAN_POINT('Ctrl Pts',(-2.60815600939102,5.90401718193932,-3.30881408541235));
#8761=CARTESIAN_POINT('Ctrl Pts',(-3.39137840827869,5.78943384860516,-2.54096498778195));
#8762=CARTESIAN_POINT('Ctrl Pts',(-3.70826592147772,5.73214218193892,-2.07753072058528));
#8763=CARTESIAN_POINT('Ctrl Pts',(-4.14174263741426,5.61755884860556,-1.05943151077492));
#8764=CARTESIAN_POINT('Ctrl Pts',(-4.25812546780629,5.56026718193889,-0.505152283069884));
#8765=CARTESIAN_POINT('Ctrl Pts',(-4.26899603338911,5.44568384860559,0.611045302667398));
#8766=CARTESIAN_POINT('Ctrl Pts',(-4.16344071207717,5.38839218193887,1.17252450979444));
#8767=CARTESIAN_POINT('Ctrl Pts',(-3.74261678141353,5.27380884860562,2.21688950738861));
#8768=CARTESIAN_POINT('Ctrl Pts',(-3.4274779112251,5.21651718193883,2.69934956768717));
#8769=CARTESIAN_POINT('Ctrl Pts',(-2.63215854609891,5.10193384860566,3.5100422341123));
#8770=CARTESIAN_POINT('Ctrl Pts',(-2.15226353660435,5.04464218193881,3.83792846364419));
#8771=CARTESIAN_POINT('Ctrl Pts',(-1.0982726926337,4.93005884860567,4.28627198125755));
#8772=CARTESIAN_POINT('Ctrl Pts',(-0.524576695510519,4.87276718193882,4.40651704719262));
#8773=CARTESIAN_POINT('Ctrl Pts',(0.630469715108076,4.75818384860567,4.41738761280318));
#8774=CARTESIAN_POINT('Ctrl Pts',(1.21136569164331,4.70089218193903,4.30797005589403));
#8775=CARTESIAN_POINT('Ctrl Pts',(2.29162232341768,4.58630884860546,3.87227932360639));
#8776=CARTESIAN_POINT('Ctrl Pts',(2.79054312598678,4.529017181939,3.5461417370364));
#8777=CARTESIAN_POINT('Ctrl Pts',(3.62870605994246,4.41443384860549,2.72335210441731));
#8778=CARTESIAN_POINT('Ctrl Pts',(3.96759100581396,4.35714218193895,2.22699635262072));
#8779=CARTESIAN_POINT('Ctrl Pts',(4.43080132509753,4.24255884860554,1.13711387449518));
#8780=CARTESIAN_POINT('Ctrl Pts',(4.55490862657983,4.18526718193866,0.544001107941954));
#8781=CARTESIAN_POINT('Ctrl Pts',(4.56577919221637,4.07068384860583,-0.649894127539557));
#8782=CARTESIAN_POINT('Ctrl Pts',(4.45249939970698,4.01339218193886,-1.25020687350361));
#8783=CARTESIAN_POINT('Ctrl Pts',(4.00194186580315,3.89880884860562,-2.36635513943533));
#8784=CARTESIAN_POINT('Ctrl Pts',(3.66480556284339,3.84151718193895,-2.88173668429245));
#8785=CARTESIAN_POINT('Ctrl Pts',(2.81454566274002,3.72693384860553,-3.74736988576655));
#8786=CARTESIAN_POINT('Ctrl Pts',(2.30172916862896,3.66964218193904,-4.09725354798759));
#8787=CARTESIAN_POINT('Ctrl Pts',(1.17595505636478,3.55505884860545,-4.57533066893367));
#8788=CARTESIAN_POINT('Ctrl Pts',(0.563425520373289,3.4977671819386,-4.70330020596852));
#8789=CARTESIAN_POINT('Ctrl Pts',(-0.669318539970923,3.38318384860588,-4.71417077162809));
#8790=CARTESIAN_POINT('Ctrl Pts',(-1.28904805536363,3.32589218193878,-4.59702874352091));
#8791=CARTESIAN_POINT('Ctrl Pts',(-2.44108795545323,3.21130884860571,-4.13160440799895));
#8792=CARTESIAN_POINT('Ctrl Pts',(-2.97293024260301,3.15401718193919,-3.78346938864651));
#8793=CARTESIAN_POINT('Ctrl Pts',(-3.86603371158577,3.03943384860528,-2.90573922106659));
#8794=CARTESIAN_POINT('Ctrl Pts',(-4.22691609016478,2.98214218193882,-2.37646198463267));
#8795=CARTESIAN_POINT('Ctrl Pts',(-4.71986001276623,2.86755884860567,-1.21479623823893));
#8796=CARTESIAN_POINT('Ctrl Pts',(-4.85169178535771,2.81026718193854,-0.582849932796644));
#8797=CARTESIAN_POINT('Ctrl Pts',(-4.86256235103931,2.69568384860595,0.688742952394343));
#8798=CARTESIAN_POINT('Ctrl Pts',(-4.74155808733321,2.638392181939,1.32788923723221));
#8799=CARTESIAN_POINT('Ctrl Pts',(-4.26126695019637,2.52380884860549,2.5158207714626));
#8800=CARTESIAN_POINT('Ctrl Pts',(-3.90213321444713,2.46651718193888,3.06412380091759));
#8801=CARTESIAN_POINT('Ctrl Pts',(-2.99693277939567,2.3519338486056,3.98469753740094));
#8802=CARTESIAN_POINT('Ctrl Pts',(-2.45119480063163,2.29464218193882,4.35657863234452));
#8803=CARTESIAN_POINT('Ctrl Pts',(-1.2536374201178,2.18005884860566,4.86438935659626));
#8804=CARTESIAN_POINT('Ctrl Pts',(-0.602274345215141,2.12276718193851,5.00008336474837));
#8805=CARTESIAN_POINT('Ctrl Pts',(0.708167364812911,2.00818384860598,5.01095393044905));
#8806=CARTESIAN_POINT('Ctrl Pts',(1.36673041909958,1.95089218193886,4.8860874311467));
#8807=CARTESIAN_POINT('Ctrl Pts',(2.59055358747315,1.83630884860562,4.39092949239261));
#8808=CARTESIAN_POINT('Ctrl Pts',(3.15531735923718,1.77901718193906,4.02079704024371));
#8809=CARTESIAN_POINT('Ctrl Pts',(4.10336136321113,1.66443384860542,3.08812633772876));
#8810=CARTESIAN_POINT('Ctrl Pts',(4.48624117452488,1.60714218193865,2.52592761663043));
#8811=CARTESIAN_POINT('Ctrl Pts',(5.00891870042567,1.49255884860583,1.29247860199682));
#8812=CARTESIAN_POINT('Ctrl Pts',(5.14847494413939,1.43526718193912,0.621698757625503));
#8813=CARTESIAN_POINT('Ctrl Pts',(5.15934550985844,1.32068384860537,-0.727591777223308));
#8814=CARTESIAN_POINT('Ctrl Pts',(5.0306167749558,1.26339218193915,-1.40557160097741));
#8815=CARTESIAN_POINT('Ctrl Pts',(4.52059203459322,1.14880884860534,-2.66528640347329));
#8816=CARTESIAN_POINT('Ctrl Pts',(4.13946086604337,1.09151718193863,-3.24651091755445));
#8817=CARTESIAN_POINT('Ctrl Pts',(3.17931989605881,0.976933848605856,-4.22202518902362));
#8818=CARTESIAN_POINT('Ctrl Pts',(2.60066043261983,0.919642181938648,-4.61590371671046));
#8819=CARTESIAN_POINT('Ctrl Pts',(1.33131978388528,0.805058848605838,-5.15344804424985));
#8820=CARTESIAN_POINT('Ctrl Pts',(0.641123170036348,0.747767181938915,-5.29686652353057));
#8821=CARTESIAN_POINT('Ctrl Pts',(-0.747016189634228,0.633183848605571,
-5.30773708926766));
#8822=CARTESIAN_POINT('Ctrl Pts',(-1.44441278286383,0.575892181939075,-5.17514611876316));
#8823=CARTESIAN_POINT('Ctrl Pts',(-2.74001921946479,0.46130884860541,-4.65025457679559));
#8824=CARTESIAN_POINT('Ctrl Pts',(-3.33770446803392,0.404017181938794,-4.25812469903555));
#8825=CARTESIAN_POINT('Ctrl Pts',(-3.83919674535392,0.346725515272242,-3.76431907311593));
#8826=CARTESIAN_POINT('Ctrl Pts',(-2.124655798183,11.0001838839337,-2.1190799629381));
#8827=CARTESIAN_POINT('Ctrl Pts',(-2.41109079938317,10.9428309226217,-1.84942416983751));
#8828=CARTESIAN_POINT('Ctrl Pts',(-2.64550594263638,10.885477961311,-1.52105845806273));
#8829=CARTESIAN_POINT('Ctrl Pts',(-2.97162798586693,10.7708333333336,-0.794830755283512));
#8830=CARTESIAN_POINT('Ctrl Pts',(-3.06332306119362,10.7135416666669,-0.397314139662748));
#8831=CARTESIAN_POINT('Ctrl Pts',(-3.08669273082211,10.5989583333331,0.407721033857582));
#8832=CARTESIAN_POINT('Ctrl Pts',(-3.01831935235521,10.5416666666666,0.814922877330024));
#8833=CARTESIAN_POINT('Ctrl Pts',(-2.728119788021,10.4270833333334,1.57659449107116));
#8834=CARTESIAN_POINT('Ctrl Pts',(-2.50637194487625,10.3697916666664,1.93074976622997));
#8835=CARTESIAN_POINT('Ctrl Pts',(-1.93991583267103,10.2552083333337,2.53025558222984));
#8836=CARTESIAN_POINT('Ctrl Pts',(-1.59540299717169,10.1979166666664,2.77534284559852));
#8837=CARTESIAN_POINT('Ctrl Pts',(-0.833671937081177,10.0833333333336,3.11615732976406));
#8838=CARTESIAN_POINT('Ctrl Pts',(-0.416738552178117,10.0260416666666,3.21171464055396));
#8839=CARTESIAN_POINT('Ctrl Pts',(0.427145446372979,9.91145833333345,3.23508431026218));
#8840=CARTESIAN_POINT('Ctrl Pts',(0.853764059103477,9.85416666666669,3.16284869617602));
#8841=CARTESIAN_POINT('Ctrl Pts',(1.65132730717562,9.73958333333332,2.85778233020993));
#8842=CARTESIAN_POINT('Ctrl Pts',(2.02194332446279,9.68229166666673,2.62503577071995));
#8843=CARTESIAN_POINT('Ctrl Pts',(2.64891940812677,9.56770833333328,2.03110939095704));
#8844=CARTESIAN_POINT('Ctrl Pts',(2.9050053877204,9.51041666666666,1.67013581324179));
#8845=CARTESIAN_POINT('Ctrl Pts',(3.26068667365192,9.39583333333334,0.872513118888943));
#8846=CARTESIAN_POINT('Ctrl Pts',(3.36010621991895,9.3385416666664,0.436162964680591));
#8847=CARTESIAN_POINT('Ctrl Pts',(3.38347588969759,9.22395833333361,-0.446569858875482));
#8848=CARTESIAN_POINT('Ctrl Pts',(3.30737803999626,9.16666666666689,-0.892605240889856));
#8849=CARTESIAN_POINT('Ctrl Pts',(2.98744487239941,9.05208333333312,-1.72606012326716));
#8850=CARTESIAN_POINT('Ctrl Pts',(2.74369959655829,8.99479166666641,-2.11313688270712));
#8851=CARTESIAN_POINT('Ctrl Pts',(2.1223029492484,8.8802083333336,-2.76758323401219));
#8852=CARTESIAN_POINT('Ctrl Pts',(1.74486862930228,8.82291666666647,-3.03466792985017));
#8853=CARTESIAN_POINT('Ctrl Pts',(0.911354300706321,8.70833333333354,-3.40521601753191));
#8854=CARTESIAN_POINT('Ctrl Pts',(0.455587377172263,8.6510416666665,-3.5084977992874));
#8855=CARTESIAN_POINT('Ctrl Pts',(-0.465994271367186,8.53645833333351,-3.53186746912954));
#8856=CARTESIAN_POINT('Ctrl Pts',(-0.93144642268745,8.47916666666683,-3.45190738381581));
#8857=CARTESIAN_POINT('Ctrl Pts',(-1.80079293934749,8.36458333333318,-3.11710741458959));
#8858=CARTESIAN_POINT('Ctrl Pts',(-2.20433044096071,8.30729166666683,-2.86236342239196));
#8859=CARTESIAN_POINT('Ctrl Pts',(-2.88624705988836,8.1927083333332,-2.21349650754444));
#8860=CARTESIAN_POINT('Ctrl Pts',(-3.1643304719878,8.13541666666656,-1.81960144535507));
#8861=CARTESIAN_POINT('Ctrl Pts',(-3.54974536140404,8.02083333333345,-0.950195482531384));
#8862=CARTESIAN_POINT('Ctrl Pts',(-3.65688937865929,7.96354166666637,-0.475011789653154));
#8863=CARTESIAN_POINT('Ctrl Pts',(-3.68025904855805,7.84895833333365,0.485418683848109));
#8864=CARTESIAN_POINT('Ctrl Pts',(-3.59643672763413,7.79166666666665,0.970287604495667));
#8865=CARTESIAN_POINT('Ctrl Pts',(-3.246769956781,7.67708333333337,1.8755257554172));
#8866=CARTESIAN_POINT('Ctrl Pts',(-2.98102724821984,7.61979166666659,2.29552399922486));
#8867=CARTESIAN_POINT('Ctrl Pts',(-2.30469006584627,7.50520833333343,3.00491088575395));
#8868=CARTESIAN_POINT('Ctrl Pts',(-1.89433426139971,7.44791666666668,3.29399301413121));
#8869=CARTESIAN_POINT('Ctrl Pts',(-0.989036664364609,7.33333333333333,3.69427470527038));
#8870=CARTESIAN_POINT('Ctrl Pts',(-0.49443620212397,7.27604166666629,3.80528095803426));
#8871=CARTESIAN_POINT('Ctrl Pts',(0.50484309631896,7.16145833333372,3.82865062798349));
#8872=CARTESIAN_POINT('Ctrl Pts',(1.00912878631411,7.10416666666678,3.74096607145172));
#8873=CARTESIAN_POINT('Ctrl Pts',(1.95025857147667,6.98958333333323,3.37643249897315));
#8874=CARTESIAN_POINT('Ctrl Pts',(2.38671755749636,6.93229166666724,3.09969107404422));
#8875=CARTESIAN_POINT('Ctrl Pts',(3.12357471161222,6.81770833333277,2.39588362415159));
#8876=CARTESIAN_POINT('Ctrl Pts',(3.42365555628099,6.76041666666712,1.96906707743673));
#8877=CARTESIAN_POINT('Ctrl Pts',(3.83880404913035,6.64583333333289,1.02787784620545));
#8878=CARTESIAN_POINT('Ctrl Pts',(3.95367253741186,6.58854166666688,0.51386061458762));
#8879=CARTESIAN_POINT('Ctrl Pts',(3.97704220740629,6.47395833333313,-0.524267508782646));
#8880=CARTESIAN_POINT('Ctrl Pts',(3.88549541526866,6.41666666666645,-1.04796996813959));
#8881=CARTESIAN_POINT('Ctrl Pts',(3.50609504116593,6.30208333333356,-2.02499138752914));
#8882=CARTESIAN_POINT('Ctrl Pts',(3.2183548998624,6.24479166666656,-2.47791111577681));
#8883=CARTESIAN_POINT('Ctrl Pts',(2.48707718246311,6.13020833333345,-3.24223853746153));
#8884=CARTESIAN_POINT('Ctrl Pts',(2.04379989346725,6.07291666666717,-3.55331809843599));
#8885=CARTESIAN_POINT('Ctrl Pts',(1.06671902805278,5.95833333333284,-3.9833333929851));
#8886=CARTESIAN_POINT('Ctrl Pts',(0.533285027040294,5.90104166666655,-4.10206411679133));
#8887=CARTESIAN_POINT('Ctrl Pts',(-0.543691921235359,5.78645833333346,-4.12543378682723));
#8888=CARTESIAN_POINT('Ctrl Pts',(-1.08681114997705,5.72916666666705,-4.03002475908303));
#8889=CARTESIAN_POINT('Ctrl Pts',(-2.0997242035696,5.61458333333296,-3.63575758336128));
#8890=CARTESIAN_POINT('Ctrl Pts',(-2.56910467406188,5.55729166666709,-3.33701872567955));
#8891=CARTESIAN_POINT('Ctrl Pts',(-3.36090236330622,5.44270833333292,-2.57827074077566));
#8892=CARTESIAN_POINT('Ctrl Pts',(-3.68298064059524,5.38541666666669,-2.11853270949184));
#8893=CARTESIAN_POINT('Ctrl Pts',(-4.12786273683561,5.27083333333332,-1.10556020990605));
#8894=CARTESIAN_POINT('Ctrl Pts',(-4.25045569617289,5.21354166666665,-0.552709439489368));
#8895=CARTESIAN_POINT('Ctrl Pts',(-4.27382536624608,5.09895833333335,0.563116333684488));
#8896=CARTESIAN_POINT('Ctrl Pts',(-4.17455410289751,5.04166666666663,1.12565233181968));
#8897=CARTESIAN_POINT('Ctrl Pts',(-3.76542012555652,4.92708333333338,2.17445701960491));
#8898=CARTESIAN_POINT('Ctrl Pts',(-3.45568255149002,4.86979166666659,2.66029823235588));
#8899=CARTESIAN_POINT('Ctrl Pts',(-2.6694642990949,4.75520833333342,3.47956618914197));
#8900=CARTESIAN_POINT('Ctrl Pts',(-2.19326552550957,4.69791666666658,3.81264318275876));
#8901=CARTESIAN_POINT('Ctrl Pts',(-1.14440139176617,4.58333333333343,4.27239208068185));
#8902=CARTESIAN_POINT('Ctrl Pts',(-0.572133851929879,4.52604166666658,4.39884727555618));
#8903=CARTESIAN_POINT('Ctrl Pts',(0.582540746125043,4.41145833333343,4.42221694566319));
#8904=CARTESIAN_POINT('Ctrl Pts',(1.16449351366757,4.35416666666679,4.31908344671154));
#8905=CARTESIAN_POINT('Ctrl Pts',(2.24918983563495,4.23958333333322,3.89508266775222));
#8906=CARTESIAN_POINT('Ctrl Pts',(2.75149179065353,4.18229166666676,3.57434637729919));
#8907=CARTESIAN_POINT('Ctrl Pts',(3.59823001497408,4.06770833333325,2.76065785741543));
#8908=CARTESIAN_POINT('Ctrl Pts',(3.94230572492611,4.01041666666671,2.26799834152485));
#8909=CARTESIAN_POINT('Ctrl Pts',(4.41692142452426,3.8958333333333,1.18324257362874));
#8910=CARTESIAN_POINT('Ctrl Pts',(4.54723885494094,3.83854166666642,0.591558264361257));
#8911=CARTESIAN_POINT('Ctrl Pts',(4.57060852507883,3.72395833333359,-0.601965158556466));
#8912=CARTESIAN_POINT('Ctrl Pts',(4.46361279052205,3.66666666666662,-1.20333469552689));
#8913=CARTESIAN_POINT('Ctrl Pts',(4.02474520995143,3.55208333333339,-2.32392265165357));
#8914=CARTESIAN_POINT('Ctrl Pts',(3.69301020310442,3.49479166666671,-2.84268534895739));
#8915=CARTESIAN_POINT('Ctrl Pts',(2.85185141573989,3.38020833333329,-3.71689384079999));
#8916=CARTESIAN_POINT('Ctrl Pts',(2.34273115753217,3.3229166666668,-4.07196826709743));
#8917=CARTESIAN_POINT('Ctrl Pts',(1.22208375549926,3.20833333333321,-4.56145076836271));
#8918=CARTESIAN_POINT('Ctrl Pts',(0.610982676792531,3.15104166666636,-4.6956304343271));
#8919=CARTESIAN_POINT('Ctrl Pts',(-0.621389570987771,3.03645833333365,-4.71900010449308));
#8920=CARTESIAN_POINT('Ctrl Pts',(-1.24217587738614,2.97916666666654,-4.60814213433379));
#8921=CARTESIAN_POINT('Ctrl Pts',(-2.39865546767225,2.86458333333347,-4.15440775214941));
#8922=CARTESIAN_POINT('Ctrl Pts',(-2.93387890726637,2.80729166666695,-3.81167402890586));
#8923=CARTESIAN_POINT('Ctrl Pts',(-3.83555766662078,2.69270833333305,-2.94304497406814));
#8924=CARTESIAN_POINT('Ctrl Pts',(-4.20163080927273,2.63541666666658,-2.41746397353493));
#8925=CARTESIAN_POINT('Ctrl Pts',(-4.70598011219716,2.52083333333343,-1.26092493737436));
#8926=CARTESIAN_POINT('Ctrl Pts',(-4.84402201371418,2.4635416666663,-0.630407089215845));
#8927=CARTESIAN_POINT('Ctrl Pts',(-4.86739168390641,2.34895833333371,0.64081398341115));
#8928=CARTESIAN_POINT('Ctrl Pts',(-4.75267147814405,2.29166666666676,1.28101705925391));
#8929=CARTESIAN_POINT('Ctrl Pts',(-4.28407029434887,2.17708333333325,2.47338828368244));
#8930=CARTESIAN_POINT('Ctrl Pts',(-3.93033785470491,2.11979166666664,3.0250724655795));
#8931=CARTESIAN_POINT('Ctrl Pts',(-3.0342385323988,2.00520833333337,3.95422149243741));
#8932=CARTESIAN_POINT('Ctrl Pts',(-2.49219678953305,1.94791666666658,4.33129335145034));
#8933=CARTESIAN_POINT('Ctrl Pts',(-1.29976611925407,1.83333333333343,4.85050945602931));
#8934=CARTESIAN_POINT('Ctrl Pts',(-0.6498315016342,1.77604166666627,4.99241359310244));
#8935=CARTESIAN_POINT('Ctrl Pts',(0.660238395829575,1.66145833333374,5.01578326331855));
#8936=CARTESIAN_POINT('Ctrl Pts',(1.31985824112059,1.60416666666663,4.89720082195578));
#8937=CARTESIAN_POINT('Ctrl Pts',(2.54812109969368,1.48958333333338,4.41373283654687));
#8938=CARTESIAN_POINT('Ctrl Pts',(3.1162660238978,1.43229166666683,4.04900168050008));
#8939=CARTESIAN_POINT('Ctrl Pts',(4.07288531824889,1.31770833333318,3.1254320907333));
#8940=CARTESIAN_POINT('Ctrl Pts',(4.460955893629,1.26041666666641,2.56692960553103));
#8941=CARTESIAN_POINT('Ctrl Pts',(4.99503879986042,1.1458333333336,1.33860730113391));
#8942=CARTESIAN_POINT('Ctrl Pts',(5.14080517249185,1.08854166666688,0.669255914044516));
#8943=CARTESIAN_POINT('Ctrl Pts',(5.16417484272955,0.973958333333134,-0.679662808239928));
#8944=CARTESIAN_POINT('Ctrl Pts',(5.04173016576313,0.916666666666909,-1.35869942299763));
#8945=CARTESIAN_POINT('Ctrl Pts',(4.54339537874923,0.8020833333331,-2.62285391569459));
#8946=CARTESIAN_POINT('Ctrl Pts',(4.16766550629842,0.744791666666392,-3.20745958221381));
#8947=CARTESIAN_POINT('Ctrl Pts',(3.21662564906467,0.630208333333619,-4.19154914406263));
#8948=CARTESIAN_POINT('Ctrl Pts',(2.6416624215197,0.572916666666411,-4.59061843581319));
#8949=CARTESIAN_POINT('Ctrl Pts',(1.3774484830231,0.4583333333336,-5.13956814368599));
#8950=CARTESIAN_POINT('Ctrl Pts',(0.688680326455284,0.401041666666677,-5.28919675188146));
#8951=CARTESIAN_POINT('Ctrl Pts',(-0.69908722065077,0.286458333333334,-5.31256642214034));
#8952=CARTESIAN_POINT('Ctrl Pts',(-1.39754060488348,0.229166666666838,-5.1862595095691));
#8953=CARTESIAN_POINT('Ctrl Pts',(-2.69758673168668,0.114583333333173,-4.67305792095299));
#8954=CARTESIAN_POINT('Ctrl Pts',(-3.29865313262765,0.0572916666665569,
-4.28632933922004));
#8955=CARTESIAN_POINT('Ctrl Pts',(-3.80443305520312,5.20417042793042E-15,
-3.79707426974638));
#8956=CARTESIAN_POINT('Ctrl Pts',(-2.08987834946245,10.6534583686615,-2.15182055112134));
#8957=CARTESIAN_POINT('Ctrl Pts',(-2.38060364826779,10.5961054073494,-1.88672201271739));
#8958=CARTESIAN_POINT('Ctrl Pts',(-2.62021456065169,10.5387524460388,-1.5620577045283));
#8959=CARTESIAN_POINT('Ctrl Pts',(-2.9577480852525,10.4241078180613,-0.840959454398505));
#8960=CARTESIAN_POINT('Ctrl Pts',(-3.05565328959838,10.3668161513947,-0.444871296083357));
#8961=CARTESIAN_POINT('Ctrl Pts',(-3.09152206364091,10.2522328180609,0.359792064875797));
#8962=CARTESIAN_POINT('Ctrl Pts',(-3.02943274321019,10.1949411513944,0.768050699368431));
#8963=CARTESIAN_POINT('Ctrl Pts',(-2.75092313212936,10.0803578180611,1.53416200327429));
#8964=CARTESIAN_POINT('Ctrl Pts',(-2.53457658516751,10.0230661513941,1.89169843092347));
#8965=CARTESIAN_POINT('Ctrl Pts',(-1.97722158564067,9.90848281806141,2.49977953723472));
#8966=CARTESIAN_POINT('Ctrl Pts',(-1.6364049860914,9.8511911513942,2.75005756474531));
#8967=CARTESIAN_POINT('Ctrl Pts',(-0.879800636199156,9.73660781806133,3.10227742915614));
#8968=CARTESIAN_POINT('Ctrl Pts',(-0.46429570859848,9.67931615139432,3.2040448689519));
#8969=CARTESIAN_POINT('Ctrl Pts',(0.379216477390949,9.56473281806121,3.2399136430878));
#8970=CARTESIAN_POINT('Ctrl Pts',(0.806891881139562,9.50744115139445,3.17396208702488));
#8971=CARTESIAN_POINT('Ctrl Pts',(1.60889481938107,9.39285781806108,2.8805856743244));
#8972=CARTESIAN_POINT('Ctrl Pts',(1.98289198915187,9.33556615139449,2.65324041100648));
#8973=CARTESIAN_POINT('Ctrl Pts',(2.61844336313606,9.22098281806105,2.06841514393141));
#8974=CARTESIAN_POINT('Ctrl Pts',(2.87972010686153,9.16369115139443,1.71113780215899));
#8975=CARTESIAN_POINT('Ctrl Pts',(3.24680677304967,9.0491078180611,0.918641818009435));
#8976=CARTESIAN_POINT('Ctrl Pts',(3.35243644831083,8.99181615139416,0.483720121100777));
#8977=CARTESIAN_POINT('Ctrl Pts',(3.38830522252928,8.87723281806137,-0.398640889893273));
#8978=CARTESIAN_POINT('Ctrl Pts',(3.31849143083958,8.81994115139465,-0.845733062923796));
#8979=CARTESIAN_POINT('Ctrl Pts',(3.01024821651943,8.70535781806088,-1.68362763547476));
#8980=CARTESIAN_POINT('Ctrl Pts',(2.77190423684068,8.64806615139417,-2.0740855473923));
#8981=CARTESIAN_POINT('Ctrl Pts',(2.15960870222691,8.53348281806136,-2.73710718902539));
#8982=CARTESIAN_POINT('Ctrl Pts',(1.78587061821714,8.47619115139423,-3.00938264898613));
#8983=CARTESIAN_POINT('Ctrl Pts',(0.957482999829145,8.36160781806131,-3.39133611693482));
#8984=CARTESIAN_POINT('Ctrl Pts',(0.503144533592307,8.30431615139426,-3.50082802767378));
#8985=CARTESIAN_POINT('Ctrl Pts',(-0.418065302384836,8.18973281806127,-3.53669680196673));
#8986=CARTESIAN_POINT('Ctrl Pts',(-0.884574244719486,8.1324411513946,-3.4630207746542));
#8987=CARTESIAN_POINT('Ctrl Pts',(-1.75836045155699,8.01785781806094,-3.13991075871454));
#8988=CARTESIAN_POINT('Ctrl Pts',(-2.16527910564236,7.96056615139459,-2.89056806267063));
#8989=CARTESIAN_POINT('Ctrl Pts',(-2.85577101490508,7.84598281806096,-2.25080226052668));
#8990=CARTESIAN_POINT('Ctrl Pts',(-3.13904519111934,7.78869115139432,-1.8606034342679));
#8991=CARTESIAN_POINT('Ctrl Pts',(-3.53586546081137,7.67410781806122,-0.996324181656243));
#8992=CARTESIAN_POINT('Ctrl Pts',(-3.64921960704095,7.61681615139413,-0.52256894607304));
#8993=CARTESIAN_POINT('Ctrl Pts',(-3.68508838139996,7.50223281806141,0.437489714865601));
#8994=CARTESIAN_POINT('Ctrl Pts',(-3.60755011846799,7.44494115139464,0.923415426526065));
#8995=CARTESIAN_POINT('Ctrl Pts',(-3.26957330091048,7.33035781806089,1.83309326762834));
#8996=CARTESIAN_POINT('Ctrl Pts',(-3.00923188849514,7.27306615139411,2.25647266390339));
#8997=CARTESIAN_POINT('Ctrl Pts',(-2.34199581883187,7.15848281806142,2.9744348407738));
#8998=CARTESIAN_POINT('Ctrl Pts',(-1.93533625031079,7.10119115139444,3.26870773325855));
#8999=CARTESIAN_POINT('Ctrl Pts',(-1.03516536349122,6.98660781806109,3.68039480468192));
#9000=CARTESIAN_POINT('Ctrl Pts',(-0.541993358543724,6.92931615139405,3.79761118641148));
#9001=CARTESIAN_POINT('Ctrl Pts',(0.45691412733632,6.81473281806148,3.83347996082984));
#9002=CARTESIAN_POINT('Ctrl Pts',(0.962256608343087,6.75744115139454,3.75207946228173));
#9003=CARTESIAN_POINT('Ctrl Pts',(1.90782608368924,6.64285781806099,3.39923584310647));
#9004=CARTESIAN_POINT('Ctrl Pts',(2.34766622217201,6.585566151395,3.12789571431651));
#9005=CARTESIAN_POINT('Ctrl Pts',(3.09309866663495,6.47098281806054,2.4331893771402));
#9006=CARTESIAN_POINT('Ctrl Pts',(3.39837027540469,6.41369115139488,2.01006906634609));
#9007=CARTESIAN_POINT('Ctrl Pts',(3.82492414854553,6.29910781806065,1.07400654533378));
#9008=CARTESIAN_POINT('Ctrl Pts',(3.94600276578516,6.24181615139464,0.561417771007294));
#9009=CARTESIAN_POINT('Ctrl Pts',(3.98187154025657,6.1272328180609,-0.476338539799928));
#9010=CARTESIAN_POINT('Ctrl Pts',(3.89660880609501,6.06994115139421,-1.00109779016719));
#9011=CARTESIAN_POINT('Ctrl Pts',(3.52889838530292,5.95535781806132,-1.98255889974307));
#9012=CARTESIAN_POINT('Ctrl Pts',(3.24655954013207,5.89806615139432,-2.43885978044999));
#9013=CARTESIAN_POINT('Ctrl Pts',(2.52438293545435,5.78348281806122,-3.21176249248673));
#9014=CARTESIAN_POINT('Ctrl Pts',(2.08480188237509,5.72619115139493,-3.52803281755643));
#9015=CARTESIAN_POINT('Ctrl Pts',(1.11284772718263,5.6116078180606,-3.96945349240354));
#9016=CARTESIAN_POINT('Ctrl Pts',(0.580842183459787,5.55431615139431,-4.0943943451612));
#9017=CARTESIAN_POINT('Ctrl Pts',(-0.495762952252458,5.43973281806122,-4.13026311968094));
#9018=CARTESIAN_POINT('Ctrl Pts',(-1.03993897200342,5.38244115139481,-4.04113814990623));
#9019=CARTESIAN_POINT('Ctrl Pts',(-2.05729171578477,5.26785781806072,-3.65856092750142));
#9020=CARTESIAN_POINT('Ctrl Pts',(-2.53005333873273,5.21056615139485,-3.36522336594676));
#9021=CARTESIAN_POINT('Ctrl Pts',(-3.33042631833374,5.09598281806069,-2.61557649376936));
#9022=CARTESIAN_POINT('Ctrl Pts',(-3.65769535971276,5.03869115139445,-2.1595346983984));
#9023=CARTESIAN_POINT('Ctrl Pts',(-4.11398283625697,4.92410781806109,-1.15168890903718));
#9024=CARTESIAN_POINT('Ctrl Pts',(-4.24278592453948,4.86681615139442,-0.600266595908851));
#9025=CARTESIAN_POINT('Ctrl Pts',(-4.27865469910306,4.75223281806112,0.515187364701578));
#9026=CARTESIAN_POINT('Ctrl Pts',(-4.18566749371785,4.69494115139439,1.07878015384492));
#9027=CARTESIAN_POINT('Ctrl Pts',(-3.78822346969952,4.58035781806114,2.13202453182121));
#9028=CARTESIAN_POINT('Ctrl Pts',(-3.48388719175493,4.52306615139435,2.62124689702459));
#9029=CARTESIAN_POINT('Ctrl Pts',(-2.70677005209088,4.40848281806118,3.44909014417165));
#9030=CARTESIAN_POINT('Ctrl Pts',(-2.2342675144148,4.35119115139434,3.78735790187333));
#9031=CARTESIAN_POINT('Ctrl Pts',(-1.19053009089864,4.2366078180612,4.25851218010615));
#9032=CARTESIAN_POINT('Ctrl Pts',(-0.61969100834924,4.17931615139434,4.39117750391975));
#9033=CARTESIAN_POINT('Ctrl Pts',(0.53461177714201,4.06473281806119,4.42704627852319));
#9034=CARTESIAN_POINT('Ctrl Pts',(1.11762133569182,4.00744115139456,4.33019683752905));
#9035=CARTESIAN_POINT('Ctrl Pts',(2.20675734785223,3.89285781806098,3.91788601189805));
#9036=CARTESIAN_POINT('Ctrl Pts',(2.71244045532029,3.83556615139452,3.60255101756198));
#9037=CARTESIAN_POINT('Ctrl Pts',(3.56775397000571,3.72098281806102,2.79796361041354));
#9038=CARTESIAN_POINT('Ctrl Pts',(3.91702044403826,3.66369115139447,2.30900033042897));
#9039=CARTESIAN_POINT('Ctrl Pts',(4.40304152395098,3.54910781806106,1.22937127276231));
#9040=CARTESIAN_POINT('Ctrl Pts',(4.53956908330205,3.49181615139418,0.63911542078056));
#9041=CARTESIAN_POINT('Ctrl Pts',(4.5754378579413,3.37723281806136,-0.554036189573376));
#9042=CARTESIAN_POINT('Ctrl Pts',(4.47472618133712,3.31994115139439,-1.15646251755018));
#9043=CARTESIAN_POINT('Ctrl Pts',(4.0475485540997,3.20535781806115,-2.28149016387182));
#9044=CARTESIAN_POINT('Ctrl Pts',(3.72121484336545,3.14806615139448,-2.80363401362233));
#9045=CARTESIAN_POINT('Ctrl Pts',(2.88915716873977,3.03348281806106,-3.68641779583343));
#9046=CARTESIAN_POINT('Ctrl Pts',(2.38373314643537,2.97619115139456,-4.04668298620726));
#9047=CARTESIAN_POINT('Ctrl Pts',(1.26821245463375,2.86160781806097,-4.54757086779175));
#9048=CARTESIAN_POINT('Ctrl Pts',(0.658539833211772,2.80431615139412,-4.68796066268569));
#9049=CARTESIAN_POINT('Ctrl Pts',(-0.573460602004618,2.68973281806141,-4.72382943735807));
#9050=CARTESIAN_POINT('Ctrl Pts',(-1.19530369940865,2.6324411513943,-4.61925552514667));
#9051=CARTESIAN_POINT('Ctrl Pts',(-2.35622297989128,2.51785781806124,-4.17721109629987));
#9052=CARTESIAN_POINT('Ctrl Pts',(-2.89482757192974,2.46056615139471,-3.83987866916521));
#9053=CARTESIAN_POINT('Ctrl Pts',(-3.8050816216558,2.34598281806081,-2.98035072706969));
#9054=CARTESIAN_POINT('Ctrl Pts',(-4.17634552838067,2.28869115139434,-2.4584659624372));
#9055=CARTESIAN_POINT('Ctrl Pts',(-4.6921002116281,2.1741078180612,-1.30705363650978));
#9056=CARTESIAN_POINT('Ctrl Pts',(-4.83635224207065,2.11681615139406,-0.677964245635046));
#9057=CARTESIAN_POINT('Ctrl Pts',(-4.87222101677351,2.00223281806147,0.592885014427957));
#9058=CARTESIAN_POINT('Ctrl Pts',(-4.76378486895489,1.94494115139452,1.23414488127561));
#9059=CARTESIAN_POINT('Ctrl Pts',(-4.30687363850137,1.83035781806102,2.43095579590228));
#9060=CARTESIAN_POINT('Ctrl Pts',(-3.95854249496268,1.77306615139441,2.98602113024142));
#9061=CARTESIAN_POINT('Ctrl Pts',(-3.07154428540192,1.65848281806113,3.92374544747388));
#9062=CARTESIAN_POINT('Ctrl Pts',(-2.53319877843447,1.60119115139435,4.30600807055617));
#9063=CARTESIAN_POINT('Ctrl Pts',(-1.34589481839034,1.48660781806119,4.83662955546236));
#9064=CARTESIAN_POINT('Ctrl Pts',(-0.697388658053259,1.42931615139403,4.9847438214565));
#9065=CARTESIAN_POINT('Ctrl Pts',(0.61230942684624,1.3147328180615,5.02061259618806));
#9066=CARTESIAN_POINT('Ctrl Pts',(1.27298606314159,1.25744115139439,4.90831421276487));
#9067=CARTESIAN_POINT('Ctrl Pts',(2.50568861191421,1.14285781806115,4.43653618070112));
#9068=CARTESIAN_POINT('Ctrl Pts',(3.07721468855841,1.08556615139459,4.07720632075644));
#9069=CARTESIAN_POINT('Ctrl Pts',(4.04240927328666,0.970982818060947,3.16273784373784));
#9070=CARTESIAN_POINT('Ctrl Pts',(4.43567061273313,0.913691151394175,2.60793159443164));
#9071=CARTESIAN_POINT('Ctrl Pts',(4.98115889929517,0.79910781806136,1.384736000271));
#9072=CARTESIAN_POINT('Ctrl Pts',(5.13313540084431,0.741816151394642,0.716813070463529));
#9073=CARTESIAN_POINT('Ctrl Pts',(5.16900417560066,0.627232818060896,-0.631733839256547));
#9074=CARTESIAN_POINT('Ctrl Pts',(5.05284355657047,0.569941151394671,-1.31182724501786));
#9075=CARTESIAN_POINT('Ctrl Pts',(4.56619872290524,0.455357818060863,-2.5804214279159));
#9076=CARTESIAN_POINT('Ctrl Pts',(4.19587014655347,0.398066151394155,-3.16840824687318));
#9077=CARTESIAN_POINT('Ctrl Pts',(3.25393140207052,0.283482818061382,-4.16107309910165));
#9078=CARTESIAN_POINT('Ctrl Pts',(2.68266441041957,0.226191151394174,-4.56533315491593));
#9079=CARTESIAN_POINT('Ctrl Pts',(1.42357718216092,0.111607818061363,-5.12568824312213));
#9080=CARTESIAN_POINT('Ctrl Pts',(0.736237482874218,0.0543161513944401,
-5.28152698023234));
#9081=CARTESIAN_POINT('Ctrl Pts',(-0.651158251667311,-0.0602671819389035,
-5.31739575501303));
#9082=CARTESIAN_POINT('Ctrl Pts',(-1.35066842690312,-0.117558848605399,
-5.19737290037505));
#9083=CARTESIAN_POINT('Ctrl Pts',(-2.65515424390857,-0.232142181939065,
-4.69586126511038));
#9084=CARTESIAN_POINT('Ctrl Pts',(-3.25960179722137,-0.28943384860568,-4.31453397940454));
#9085=CARTESIAN_POINT('Ctrl Pts',(-3.76966936505231,-0.346725515272232,
-3.82982946637684));
#9086=CARTESIAN_POINT('Ctrl Pts',(-2.32979046439652,10.6534583686615,-2.40665810101083));
#9087=CARTESIAN_POINT('Ctrl Pts',(-2.65390980629198,10.5961054073494,-2.1101216920847));
#9088=CARTESIAN_POINT('Ctrl Pts',(-2.92064337015263,10.5387524460388,-1.74738451990478));
#9089=CARTESIAN_POINT('Ctrl Pts',(-3.29576381367816,10.4241078180613,-0.942666738728406));
#9090=CARTESIAN_POINT('Ctrl Pts',(-3.40413627693083,10.3668161513947,-0.501072825334149));
#9091=CARTESIAN_POINT('Ctrl Pts',(-3.44272956946446,10.2522328180609,0.39517980573707));
#9092=CARTESIAN_POINT('Ctrl Pts',(-3.37289643675743,10.1949411513944,0.849485922498689));
#9093=CARTESIAN_POINT('Ctrl Pts',(-3.06185425628309,10.0803578180611,1.70125730657109));
#9094=CARTESIAN_POINT('Ctrl Pts',(-2.82073175110235,10.0230661513941,2.0983726319291));
#9095=CARTESIAN_POINT('Ctrl Pts',(-2.2005398830606,9.90848281806141,2.77314365775904));
#9096=CARTESIAN_POINT('Ctrl Pts',(-1.82168709441022,9.8511911513942,3.05050647003645));
#9097=CARTESIAN_POINT('Ctrl Pts',(-0.98150792048159,9.73660781806133,3.44029315760313));
#9098=CARTESIAN_POINT('Ctrl Pts',(-0.520497237899657,9.67931615139432,3.55252785628273));
#9099=CARTESIAN_POINT('Ctrl Pts',(0.41460421830261,9.56473281806121,3.59112114891296));
#9100=CARTESIAN_POINT('Ctrl Pts',(0.888327104224163,9.50744115139445,3.51742578058933));
#9101=CARTESIAN_POINT('Ctrl Pts',(1.77599012272354,9.39285781806108,3.19151679846092));
#9102=CARTESIAN_POINT('Ctrl Pts',(2.18956619012306,9.33556615139449,2.93939557697384));
#9103=CARTESIAN_POINT('Ctrl Pts',(2.89180748369484,9.22098281806105,2.29173344131881));
#9104=CARTESIAN_POINT('Ctrl Pts',(3.18016901213384,9.16369115139443,1.8964199105197));
#9105=CARTESIAN_POINT('Ctrl Pts',(3.58482250151549,9.0491078180611,1.02034910224998));
#9106=CARTESIAN_POINT('Ctrl Pts',(3.70091943564033,8.99181615139416,0.539921650446381));
#9107=CARTESIAN_POINT('Ctrl Pts',(3.73951272835577,8.87723281806137,-0.434028630849363));
#9108=CARTESIAN_POINT('Ctrl Pts',(3.66195512441954,8.81994115139465,-0.927168285967855));
#9109=CARTESIAN_POINT('Ctrl Pts',(3.32117934064045,8.70535781806088,-1.85072293885776));
#9110=CARTESIAN_POINT('Ctrl Pts',(3.05805940283662,8.64806615139417,-2.28075974833291));
#9111=CARTESIAN_POINT('Ctrl Pts',(2.38292699958574,8.53348281806136,-3.01047130961474));
#9112=CARTESIAN_POINT('Ctrl Pts',(1.97115272661516,8.47619115139423,-3.30983155424184));
#9113=CARTESIAN_POINT('Ctrl Pts',(1.05919028403238,8.36160781806131,-3.72935184541724));
#9114=CARTESIAN_POINT('Ctrl Pts',(0.559346062977529,8.30431615139426,-3.8493110150021));
#9115=CARTESIAN_POINT('Ctrl Pts',(-0.453453043380547,8.18973281806127,-3.8879043077944));
#9116=CARTESIAN_POINT('Ctrl Pts',(-0.966009467727636,8.1324411513946,-3.80648446824784));
#9117=CARTESIAN_POINT('Ctrl Pts',(-1.92545575497591,8.01785781806094,-3.45084188282187));
#9118=CARTESIAN_POINT('Ctrl Pts',(-2.37195330655562,7.96056615139459,-3.17672322869252));
#9119=CARTESIAN_POINT('Ctrl Pts',(-3.12913513552178,7.84598281806096,-2.47412055785955));
#9120=CARTESIAN_POINT('Ctrl Pts',(-3.43949409635991,7.78869115139432,-2.04588554269906));
#9121=CARTESIAN_POINT('Ctrl Pts',(-3.87388118930893,7.67410781806122,-1.09803146582633));
#9122=CARTESIAN_POINT('Ctrl Pts',(-3.9977025943682,7.61681615139413,-0.578770475493801));
#9123=CARTESIAN_POINT('Ctrl Pts',(-4.03629588722871,7.50223281806141,0.472877455896854));
#9124=CARTESIAN_POINT('Ctrl Pts',(-3.95101381207413,7.44494115139464,1.00485064950196));
#9125=CARTESIAN_POINT('Ctrl Pts',(-3.58050442500531,7.33035781806089,2.00018857107951));
#9126=CARTESIAN_POINT('Ctrl Pts',(-3.29538705454006,7.27306615139411,2.46314686479214));
#9127=CARTESIAN_POINT('Ctrl Pts',(-2.56531411614172,7.15848281806142,3.24779896141502));
#9128=CARTESIAN_POINT('Ctrl Pts',(-2.12061835877177,7.10119115139444,3.5691566384858));
#9129=CARTESIAN_POINT('Ctrl Pts',(-1.13687264763148,6.98660781806109,4.01841053319279));
#9130=CARTESIAN_POINT('Ctrl Pts',(-0.598194887996293,6.92931615139405,4.14609417373796));
#9131=CARTESIAN_POINT('Ctrl Pts',(0.492301868399383,6.81473281806148,4.18468746665935));
#9132=CARTESIAN_POINT('Ctrl Pts',(1.04369183128993,6.75744115139454,4.09554315589853));
#9133=CARTESIAN_POINT('Ctrl Pts',(2.07492138716947,6.64285781806099,3.71016696719063));
#9134=CARTESIAN_POINT('Ctrl Pts',(2.55434042303921,6.585566151395,3.41405088038211));
#9135=CARTESIAN_POINT('Ctrl Pts',(3.36646278729771,6.47098281806054,2.65650767442937));
#9136=CARTESIAN_POINT('Ctrl Pts',(3.69881918061998,6.41369115139488,2.19535117483371));
#9137=CARTESIAN_POINT('Ctrl Pts',(4.16293987706837,6.29910781806065,1.1757138294474));
#9138=CARTESIAN_POINT('Ctrl Pts',(4.29448575311062,6.24181615139464,0.617619300488533));
#9139=CARTESIAN_POINT('Ctrl Pts',(4.3330790460871,6.1272328180609,-0.511726280891663));
#9140=CARTESIAN_POINT('Ctrl Pts',(4.24007249972198,6.06994115139421,-1.0825330130876));
#9141=CARTESIAN_POINT('Ctrl Pts',(3.8398295093769,5.95535781806132,-2.14965420324974));
#9142=CARTESIAN_POINT('Ctrl Pts',(3.53271470621635,5.89806615139432,-2.64553398129709));
#9143=CARTESIAN_POINT('Ctrl Pts',(2.74770123272482,5.78348281806122,-3.48512661316959));
#9144=CARTESIAN_POINT('Ctrl Pts',(2.27008399088731,5.72619115139493,-3.82848172276042));
#9145=CARTESIAN_POINT('Ctrl Pts',(1.21455501127165,5.6116078180606,-4.30746922093769));
#9146=CARTESIAN_POINT('Ctrl Pts',(0.637043712966868,5.55431615139431,-4.44287733248579));
#9147=CARTESIAN_POINT('Ctrl Pts',(-0.531150693370039,5.43973281806122,-4.48147062551234));
#9148=CARTESIAN_POINT('Ctrl Pts',(-1.12137419490063,5.38244115139481,-4.38460184354212));
#9149=CARTESIAN_POINT('Ctrl Pts',(-2.22438701931463,5.26785781806072,-3.96949205156649));
#9150=CARTESIAN_POINT('Ctrl Pts',(-2.73672753956158,5.21056615139485,-3.651378532048));
#9151=CARTESIAN_POINT('Ctrl Pts',(-3.60379043903486,5.09598281806069,-2.83889479102288));
#9152=CARTESIAN_POINT('Ctrl Pts',(-3.95814426490714,5.03869115139445,-2.34481680693236));
#9153=CARTESIAN_POINT('Ctrl Pts',(-4.45199856480073,4.92410781806109,-1.25339619310446));
#9154=CARTESIAN_POINT('Ctrl Pts',(-4.59126891186371,4.86681615139442,-0.656468125439367));
#9155=CARTESIAN_POINT('Ctrl Pts',(-4.62986220493482,4.75223281806112,0.550575105842595));
#9156=CARTESIAN_POINT('Ctrl Pts',(-4.52913118736181,4.69494115139439,1.1602153767205));
#9157=CARTESIAN_POINT('Ctrl Pts',(-4.09915459375653,4.58035781806114,2.2991198353727));
#9158=CARTESIAN_POINT('Ctrl Pts',(-3.77004235787144,4.52306615139435,2.82792109783747));
#9159=CARTESIAN_POINT('Ctrl Pts',(-2.93008834932913,4.40848281806118,3.72245426488873));
#9160=CARTESIAN_POINT('Ctrl Pts',(-2.41954962296883,4.35119115139434,4.08780680705904));
#9161=CARTESIAN_POINT('Ctrl Pts',(-1.29223737494584,4.2366078180612,4.59652790865858));
#9162=CARTESIAN_POINT('Ctrl Pts',(-0.675892537901207,4.17931615139434,4.73966049124289));
#9163=CARTESIAN_POINT('Ctrl Pts',(0.569999518304482,4.06473281806119,4.77825378435605));
#9164=CARTESIAN_POINT('Ctrl Pts',(1.19905655854802,4.00744115139456,4.67366053118015));
#9165=CARTESIAN_POINT('Ctrl Pts',(2.37385265142312,3.89285781806098,4.2288171359479));
#9166=CARTESIAN_POINT('Ctrl Pts',(2.91911465611821,3.83556615139452,3.88870618369294));
#9167=CARTESIAN_POINT('Ctrl Pts',(3.84111809073776,3.72098281806102,3.02128190763733));
#9168=CARTESIAN_POINT('Ctrl Pts',(4.21746934921548,3.66369115139447,2.49428243900129));
#9169=CARTESIAN_POINT('Ctrl Pts',(4.74105725251191,3.54910781806106,1.33107855679123));
#9170=CARTESIAN_POINT('Ctrl Pts',(4.88805207062498,3.49181615139418,0.695316950351842));
#9171=CARTESIAN_POINT('Ctrl Pts',(4.92664536377436,3.37723281806136,-0.589423930755165));
#9172=CARTESIAN_POINT('Ctrl Pts',(4.81818987499502,3.31994115139439,-1.23789774038871));
#9173=CARTESIAN_POINT('Ctrl Pts',(4.35847967814275,3.20535781806115,-2.44858546746038));
#9174=CARTESIAN_POINT('Ctrl Pts',(4.00737000950903,3.14806615139448,-3.01030821440669));
#9175=CARTESIAN_POINT('Ctrl Pts',(3.11247546595094,3.03348281806106,-3.95978191657904));
#9176=CARTESIAN_POINT('Ctrl Pts',(2.56901525502413,2.97619115139456,-4.34713189137729));
#9177=CARTESIAN_POINT('Ctrl Pts',(1.36991973864622,2.86160781806097,-4.88558659635986));
#9178=CARTESIAN_POINT('Ctrl Pts',(0.714741362801074,2.80431615139412,-5.0364436500079));
#9179=CARTESIAN_POINT('Ctrl Pts',(-0.608848343204429,2.68973281806141,-5.07503694319185));
#9180=CARTESIAN_POINT('Ctrl Pts',(-1.27673892223029,2.6324411513943,-4.96271921881159));
#9181=CARTESIAN_POINT('Ctrl Pts',(-2.52331828349673,2.51785781806124,-4.48814222033592));
#9182=CARTESIAN_POINT('Ctrl Pts',(-3.10150177270171,2.46056615139471,-4.12603383532024));
#9183=CARTESIAN_POINT('Ctrl Pts',(-4.0784457424138,2.34598281806081,-3.20366902426941));
#9184=CARTESIAN_POINT('Ctrl Pts',(-4.47679443354355,2.28869115139434,-2.64374807104099));
#9185=CARTESIAN_POINT('Ctrl Pts',(-5.03011594020335,2.1741078180612,-1.40876092050723));
#9186=CARTESIAN_POINT('Ctrl Pts',(-5.18483522939207,2.11681615139406,-0.734165775240769));
#9187=CARTESIAN_POINT('Ctrl Pts',(-5.22342852260808,2.00223281806147,0.628272755644193));
#9188=CARTESIAN_POINT('Ctrl Pts',(-5.10724856262497,1.94494115139452,1.31558010408276));
#9189=CARTESIAN_POINT('Ctrl Pts',(-4.61780476253225,1.83035781806102,2.59805109952221));
#9190=CARTESIAN_POINT('Ctrl Pts',(-4.24469766112837,1.77306615139441,3.1926953310021));
#9191=CARTESIAN_POINT('Ctrl Pts',(-3.29486258259099,1.65848281806113,4.19710956824316));
#9192=CARTESIAN_POINT('Ctrl Pts',(-2.71848088705236,1.60119115139435,4.60645697571289));
#9193=CARTESIAN_POINT('Ctrl Pts',(-1.44760210237368,1.48660781806119,5.17464528404378));
#9194=CARTESIAN_POINT('Ctrl Pts',(-0.753590187674045,1.42931615139403,5.33322680877775));
#9195=CARTESIAN_POINT('Ctrl Pts',(0.647697168077543,1.3147328180615,5.37182010202281));
#9196=CARTESIAN_POINT('Ctrl Pts',(1.35442128593412,1.25744115139439,5.25177790643984));
#9197=CARTESIAN_POINT('Ctrl Pts',(2.67278391554878,1.14285781806115,4.74746730472711));
#9198=CARTESIAN_POINT('Ctrl Pts',(3.28388888930855,1.08556615139459,4.36336148693201));
#9199=CARTESIAN_POINT('Ctrl Pts',(4.3157733940665,0.970982818060947,3.38605614091702));
#9200=CARTESIAN_POINT('Ctrl Pts',(4.73611951788435,0.913691151394175,2.79321370306255));
#9201=CARTESIAN_POINT('Ctrl Pts',(5.31917462788209,0.79910781806136,1.48644328424131));
#9202=CARTESIAN_POINT('Ctrl Pts',(5.48161838816491,0.741816151394642,0.773014600098004));
#9203=CARTESIAN_POINT('Ctrl Pts',(5.52021168143606,0.627232818060896,-0.667121580501539));
#9204=CARTESIAN_POINT('Ctrl Pts',(5.39630725025002,0.569941151394671,-1.39326246779836));
#9205=CARTESIAN_POINT('Ctrl Pts',(4.87712984692664,0.455357818060863,-2.7475167315625));
#9206=CARTESIAN_POINT('Ctrl Pts',(4.48202531273885,0.398066151394155,-3.37508244761294));
#9207=CARTESIAN_POINT('Ctrl Pts',(3.47724969923989,0.283482818061382,-4.43443721989186));
#9208=CARTESIAN_POINT('Ctrl Pts',(2.8679465190623,0.226191151394174,-4.86578206006134));
#9209=CARTESIAN_POINT('Ctrl Pts',(1.52528446611942,0.111607818061363,-5.46370397171486));
#9210=CARTESIAN_POINT('Ctrl Pts',(0.792439012521748,0.0543161513944402,
-5.63000996755282));
#9211=CARTESIAN_POINT('Ctrl Pts',(-0.686545992925361,-0.0602671819389035,
-5.66860326084855));
#9212=CARTESIAN_POINT('Ctrl Pts',(-1.43210364967231,-0.117558848605399,
-5.54083659405887));
#9213=CARTESIAN_POINT('Ctrl Pts',(-2.82224954756648,-0.232142181939065,
-5.00679238912752));
#9214=CARTESIAN_POINT('Ctrl Pts',(-3.46627599744854,-0.28943384860568,-4.6006891460729));
#9215=CARTESIAN_POINT('Ctrl Pts',(-4.0096885258173,-0.346725515272232,-4.08456619805421));
#9216=CARTESIAN_POINT('Ctrl Pts',(-2.36456791311707,11.0001838839337,-2.37391751282759));
#9217=CARTESIAN_POINT('Ctrl Pts',(-2.68439695740737,10.9428309226217,-2.07282384920463));
#9218=CARTESIAN_POINT('Ctrl Pts',(-2.94593475213736,10.885477961311,-1.70638527343931));
#9219=CARTESIAN_POINT('Ctrl Pts',(-3.30964371429254,10.7708333333336,-0.896538039613314));
#9220=CARTESIAN_POINT('Ctrl Pts',(-3.41180604852602,10.7135416666669,-0.453515668913589));
#9221=CARTESIAN_POINT('Ctrl Pts',(-3.4379002366457,10.5989583333331,0.443108774718904));
#9222=CARTESIAN_POINT('Ctrl Pts',(-3.36178304590245,10.5416666666666,0.896358100460257));
#9223=CARTESIAN_POINT('Ctrl Pts',(-3.03905091217473,10.4270833333334,1.74368979436799));
#9224=CARTESIAN_POINT('Ctrl Pts',(-2.79252711081109,10.3697916666664,2.13742396723561));
#9225=CARTESIAN_POINT('Ctrl Pts',(-2.16323413009096,10.2552083333337,2.80361970275416));
#9226=CARTESIAN_POINT('Ctrl Pts',(-1.78068510549046,10.1979166666664,3.07579175088966));
#9227=CARTESIAN_POINT('Ctrl Pts',(-0.935379221363662,10.0833333333336,3.45417305821104));
#9228=CARTESIAN_POINT('Ctrl Pts',(-0.472940081479242,10.0260416666666,3.56019762788479));
#9229=CARTESIAN_POINT('Ctrl Pts',(0.462533187284589,9.91145833333345,3.58629181608734));
#9230=CARTESIAN_POINT('Ctrl Pts',(0.935199282188079,9.85416666666669,3.50631238974053));
#9231=CARTESIAN_POINT('Ctrl Pts',(1.81842261051809,9.73958333333332,3.16871345434639));
#9232=CARTESIAN_POINT('Ctrl Pts',(2.22861752543397,9.68229166666673,2.91119093668731));
#9233=CARTESIAN_POINT('Ctrl Pts',(2.92228352868554,9.56770833333328,2.25442768834444));
#9234=CARTESIAN_POINT('Ctrl Pts',(3.20545429299277,9.51041666666666,1.85541792160244));
#9235=CARTESIAN_POINT('Ctrl Pts',(3.59870240211769,9.39583333333334,0.974220403129539));
#9236=CARTESIAN_POINT('Ctrl Pts',(3.70858920724845,9.3385416666664,0.492364494026195));
#9237=CARTESIAN_POINT('Ctrl Pts',(3.73468339552408,9.22395833333361,-0.481957599831572));
#9238=CARTESIAN_POINT('Ctrl Pts',(3.65084173357628,9.16666666666689,-0.974040463933888));
#9239=CARTESIAN_POINT('Ctrl Pts',(3.29837599652037,9.05208333333312,-1.8931554266502));
#9240=CARTESIAN_POINT('Ctrl Pts',(3.02985476255422,8.99479166666641,-2.31981108364774));
#9241=CARTESIAN_POINT('Ctrl Pts',(2.34562124660724,8.8802083333336,-3.04094735460153));
#9242=CARTESIAN_POINT('Ctrl Pts',(1.93015073770027,8.82291666666647,-3.33511683510577));
#9243=CARTESIAN_POINT('Ctrl Pts',(1.01306158490958,8.70833333333354,-3.74323174601444));
#9244=CARTESIAN_POINT('Ctrl Pts',(0.511788906557484,8.6510416666665,-3.85698078661577));
#9245=CARTESIAN_POINT('Ctrl Pts',(-0.501382012362897,8.53645833333351,-3.88307497495716));
#9246=CARTESIAN_POINT('Ctrl Pts',(-1.01288164569554,8.47916666666683,-3.79537107740945));
#9247=CARTESIAN_POINT('Ctrl Pts',(-1.96788824276646,8.36458333333318,-3.42803853869692));
#9248=CARTESIAN_POINT('Ctrl Pts',(-2.41100464187403,8.30729166666683,-3.14851858841386));
#9249=CARTESIAN_POINT('Ctrl Pts',(-3.159611180505,8.1927083333332,-2.43681480487731));
#9250=CARTESIAN_POINT('Ctrl Pts',(-3.46477937722837,8.13541666666656,-2.00488355378617));
#9251=CARTESIAN_POINT('Ctrl Pts',(-3.8877610899016,8.02083333333345,-1.05190276670153));
#9252=CARTESIAN_POINT('Ctrl Pts',(-4.00537236598643,7.96354166666637,-0.531213319073915));
#9253=CARTESIAN_POINT('Ctrl Pts',(-4.03146655438691,7.84895833333365,0.520806424879362));
#9254=CARTESIAN_POINT('Ctrl Pts',(-3.93990042124014,7.79166666666665,1.05172282747159));
#9255=CARTESIAN_POINT('Ctrl Pts',(-3.55770108087595,7.67708333333337,2.04262105886835));
#9256=CARTESIAN_POINT('Ctrl Pts',(-3.26718241426475,7.61979166666659,2.50219820011361));
#9257=CARTESIAN_POINT('Ctrl Pts',(-2.52800836315612,7.50520833333343,3.27827500639517));
#9258=CARTESIAN_POINT('Ctrl Pts',(-2.07961636986072,7.44791666666668,3.59444191935829));
#9259=CARTESIAN_POINT('Ctrl Pts',(-1.09074394850484,7.33333333333333,4.03229043378143));
#9260=CARTESIAN_POINT('Ctrl Pts',(-0.550637731576509,7.27604166666629,4.15376394536062));
#9261=CARTESIAN_POINT('Ctrl Pts',(0.540230837381994,7.16145833333372,4.17985813381312));
#9262=CARTESIAN_POINT('Ctrl Pts',(1.09056400926098,7.10416666666678,4.08442976506864));
#9263=CARTESIAN_POINT('Ctrl Pts',(2.11735387495688,6.98958333333323,3.68736362305719));
#9264=CARTESIAN_POINT('Ctrl Pts',(2.59339175836345,6.93229166666724,3.38584624010982));
#9265=CARTESIAN_POINT('Ctrl Pts',(3.3969388322751,6.81770833333277,2.61920192144075));
#9266=CARTESIAN_POINT('Ctrl Pts',(3.72410446149635,6.76041666666712,2.15434918592434));
#9267=CARTESIAN_POINT('Ctrl Pts',(4.17681977765313,6.64583333333289,1.12958513031907));
#9268=CARTESIAN_POINT('Ctrl Pts',(4.30215552473732,6.58854166666688,0.570062144068889));
#9269=CARTESIAN_POINT('Ctrl Pts',(4.32824971323683,6.47395833333313,-0.559655249874413));
#9270=CARTESIAN_POINT('Ctrl Pts',(4.22895910889563,6.41666666666645,-1.12940519106012));
#9271=CARTESIAN_POINT('Ctrl Pts',(3.81702616523991,6.30208333333356,-2.19208669103568));
#9272=CARTESIAN_POINT('Ctrl Pts',(3.50451006594675,6.24479166666656,-2.68458531662391));
#9273=CARTESIAN_POINT('Ctrl Pts',(2.71039547973352,6.13020833333345,-3.51560265814439));
#9274=CARTESIAN_POINT('Ctrl Pts',(2.22908200197935,6.07291666666717,-3.85376700363998));
#9275=CARTESIAN_POINT('Ctrl Pts',(1.16842631214193,5.95833333333284,-4.32134912151925));
#9276=CARTESIAN_POINT('Ctrl Pts',(0.589486556547344,5.90104166666655,-4.45054710411593));
#9277=CARTESIAN_POINT('Ctrl Pts',(-0.579079662352908,5.78645833333346,-4.47664129265863));
#9278=CARTESIAN_POINT('Ctrl Pts',(-1.16824637287424,5.72916666666705,-4.37348845271886));
#9279=CARTESIAN_POINT('Ctrl Pts',(-2.26681950709949,5.61458333333296,-3.94668870742641));
#9280=CARTESIAN_POINT('Ctrl Pts',(-2.77577887489086,5.55729166666709,-3.62317389178086));
#9281=CARTESIAN_POINT('Ctrl Pts',(-3.6342664840072,5.44270833333292,-2.80158903802911));
#9282=CARTESIAN_POINT('Ctrl Pts',(-3.98342954578962,5.38541666666669,-2.30381481802579));
#9283=CARTESIAN_POINT('Ctrl Pts',(-4.46587846537937,5.27083333333332,-1.20726749397333));
#9284=CARTESIAN_POINT('Ctrl Pts',(-4.59893868349712,5.21354166666665,-0.608910969019916));
#9285=CARTESIAN_POINT('Ctrl Pts',(-4.62503287207784,5.09895833333335,0.598504074825539));
#9286=CARTESIAN_POINT('Ctrl Pts',(-4.51801779654147,5.04166666666663,1.20708755469526));
#9287=CARTESIAN_POINT('Ctrl Pts',(-4.07635124961353,4.92708333333338,2.34155232315641));
#9288=CARTESIAN_POINT('Ctrl Pts',(-3.74183771760646,4.86979166666659,2.86697243316876));
#9289=CARTESIAN_POINT('Ctrl Pts',(-2.89278259633321,4.75520833333342,3.75293030985906));
#9290=CARTESIAN_POINT('Ctrl Pts',(-2.37854763406351,4.69791666666658,4.1130920879442));
#9291=CARTESIAN_POINT('Ctrl Pts',(-1.24610867581347,4.58333333333343,4.61040780923455));
#9292=CARTESIAN_POINT('Ctrl Pts',(-0.628335381481812,4.52604166666658,4.74733026287932));
#9293=CARTESIAN_POINT('Ctrl Pts',(0.617928487287482,4.41145833333343,4.77342445149605));
#9294=CARTESIAN_POINT('Ctrl Pts',(1.24592873652376,4.35416666666679,4.66254714036264));
#9295=CARTESIAN_POINT('Ctrl Pts',(2.41628513920584,4.23958333333322,4.20601379180208));
#9296=CARTESIAN_POINT('Ctrl Pts',(2.95816599145146,4.18229166666676,3.86050154342994));
#9297=CARTESIAN_POINT('Ctrl Pts',(3.87159413570613,4.06770833333325,2.98397615463943));
#9298=CARTESIAN_POINT('Ctrl Pts',(4.24275463010319,4.01041666666671,2.45328045009706));
#9299=CARTESIAN_POINT('Ctrl Pts',(4.75493715308532,3.8958333333333,1.28494985765777));
#9300=CARTESIAN_POINT('Ctrl Pts',(4.89572184226387,3.83854166666642,0.647759793932574));
#9301=CARTESIAN_POINT('Ctrl Pts',(4.9218160309119,3.72395833333359,-0.637352899738291));
#9302=CARTESIAN_POINT('Ctrl Pts',(4.80707648417982,3.66666666666662,-1.28476991836542));
#9303=CARTESIAN_POINT('Ctrl Pts',(4.33567633399462,3.55208333333339,-2.49101795524214));
#9304=CARTESIAN_POINT('Ctrl Pts',(3.97916536924807,3.49479166666671,-3.04935954974168));
#9305=CARTESIAN_POINT('Ctrl Pts',(3.075169712951,3.38020833333329,-3.99025796154567));
#9306=CARTESIAN_POINT('Ctrl Pts',(2.52801326612096,3.3229166666668,-4.37241717226731));
#9307=CARTESIAN_POINT('Ctrl Pts',(1.3237910395117,3.20833333333321,-4.89946649693097));
#9308=CARTESIAN_POINT('Ctrl Pts',(0.667184206381905,3.15104166666636,-5.04411342164931));
#9309=CARTESIAN_POINT('Ctrl Pts',(-0.656777312187654,3.03645833333365,-5.07020761032686));
#9310=CARTESIAN_POINT('Ctrl Pts',(-1.32361110020785,2.97916666666654,-4.95160582799841));
#9311=CARTESIAN_POINT('Ctrl Pts',(-2.56575077127763,2.86458333333347,-4.46533887618575));
#9312=CARTESIAN_POINT('Ctrl Pts',(-3.1405531080382,2.80729166666695,-4.09782919506089));
#9313=CARTESIAN_POINT('Ctrl Pts',(-4.10892178737893,2.69270833333305,-3.16636327126786));
#9314=CARTESIAN_POINT('Ctrl Pts',(-4.50207971443576,2.63541666666658,-2.60274608213879));
#9315=CARTESIAN_POINT('Ctrl Pts',(-5.04399584077227,2.52083333333343,-1.36263222137173));
#9316=CARTESIAN_POINT('Ctrl Pts',(-5.1925050010359,2.4635416666663,-0.686608618821642));
#9317=CARTESIAN_POINT('Ctrl Pts',(-5.21859918974068,2.34895833333371,0.67620172462746));
#9318=CARTESIAN_POINT('Ctrl Pts',(-5.09613517181383,2.29166666666676,1.36245228206106));
#9319=CARTESIAN_POINT('Ctrl Pts',(-4.59500141838005,2.17708333333325,2.64048358730238));
#9320=CARTESIAN_POINT('Ctrl Pts',(-4.21649302087059,2.11979166666664,3.23174666634004));
#9321=CARTESIAN_POINT('Ctrl Pts',(-3.25755682958786,2.00520833333337,4.22758561320685));
#9322=CARTESIAN_POINT('Ctrl Pts',(-2.67747889815098,1.94791666666658,4.63174225660692));
#9323=CARTESIAN_POINT('Ctrl Pts',(-1.40147340323737,1.83333333333343,5.18852518461089));
#9324=CARTESIAN_POINT('Ctrl Pts',(-0.706033031254986,1.77604166666627,5.34089658042353));
#9325=CARTESIAN_POINT('Ctrl Pts',(0.695626137060878,1.66145833333374,5.36699076915345));
#9326=CARTESIAN_POINT('Ctrl Pts',(1.40129346391331,1.60416666666663,5.24066451563091));
#9327=CARTESIAN_POINT('Ctrl Pts',(2.71521640332806,1.48958333333338,4.7246639605727));
#9328=CARTESIAN_POINT('Ctrl Pts',(3.32294022464786,1.43229166666683,4.33515684667557));
#9329=CARTESIAN_POINT('Ctrl Pts',(4.34624943902881,1.31770833333318,3.34875038791256));
#9330=CARTESIAN_POINT('Ctrl Pts',(4.76140479878007,1.26041666666641,2.75221171416214));
#9331=CARTESIAN_POINT('Ctrl Pts',(5.3330545284475,1.1458333333336,1.44031458510402));
#9332=CARTESIAN_POINT('Ctrl Pts',(5.48928815981245,1.08854166666688,0.72545744367903));
#9333=CARTESIAN_POINT('Ctrl Pts',(5.51538234856494,0.973958333333134,-0.715050549484959));
#9334=CARTESIAN_POINT('Ctrl Pts',(5.38519385944284,0.916666666666909,-1.44013464577813));
#9335=CARTESIAN_POINT('Ctrl Pts',(4.85432650277048,0.8020833333331,-2.7899492193412));
#9336=CARTESIAN_POINT('Ctrl Pts',(4.4538206724838,0.744791666666392,-3.4141337829535));
#9337=CARTESIAN_POINT('Ctrl Pts',(3.43994394623404,0.630208333333619,-4.46491326485293));
#9338=CARTESIAN_POINT('Ctrl Pts',(2.82694453016243,0.572916666666411,-4.89106734095877));
#9339=CARTESIAN_POINT('Ctrl Pts',(1.47915576698159,0.4583333333336,-5.47758387227856));
#9340=CARTESIAN_POINT('Ctrl Pts',(0.744881856102772,0.401041666666677,-5.63767973920226));
#9341=CARTESIAN_POINT('Ctrl Pts',(-0.73447496190878,0.286458333333334,-5.66377392797554));
#9342=CARTESIAN_POINT('Ctrl Pts',(-1.4789758276525,0.229166666666838,-5.52972320325324));
#9343=CARTESIAN_POINT('Ctrl Pts',(-2.86468203534475,0.114583333333173,-4.9839890449698));
#9344=CARTESIAN_POINT('Ctrl Pts',(-3.50532733285514,0.0572916666665569,
-4.5724845058884));
#9345=CARTESIAN_POINT('Ctrl Pts',(-4.04445221596811,5.20417042793042E-15,
-4.05181100142375));
#9346=CARTESIAN_POINT('',(-3.80443305520312,5.15793290147402E-15,-3.79707426974638));
#9347=CARTESIAN_POINT('Ctrl Pts',(-2.45534485149915,10.9282219455009,-1.7516666854678));
#9348=CARTESIAN_POINT('Ctrl Pts',(-2.59470810356228,10.8948562970005,-1.56864042896568));
#9349=CARTESIAN_POINT('Ctrl Pts',(-2.71374107587765,10.8614906485003,-1.3691084593084));
#9350=CARTESIAN_POINT('Ctrl Pts',(-2.97162798586693,10.7708333333336,-0.794830755283512));
#9351=CARTESIAN_POINT('Ctrl Pts',(-3.06332306119362,10.7135416666669,-0.397314139662748));
#9352=CARTESIAN_POINT('Ctrl Pts',(-3.08669273082211,10.5989583333331,0.407721033857582));
#9353=CARTESIAN_POINT('Ctrl Pts',(-3.01831935235521,10.5416666666666,0.814922877330024));
#9354=CARTESIAN_POINT('Ctrl Pts',(-2.728119788021,10.4270833333334,1.57659449107116));
#9355=CARTESIAN_POINT('Ctrl Pts',(-2.50637194487625,10.3697916666664,1.93074976622997));
#9356=CARTESIAN_POINT('Ctrl Pts',(-1.93991583267103,10.2552083333337,2.53025558222984));
#9357=CARTESIAN_POINT('Ctrl Pts',(-1.59540299717169,10.1979166666664,2.77534284559852));
#9358=CARTESIAN_POINT('Ctrl Pts',(-0.833671937081177,10.0833333333336,3.11615732976406));
#9359=CARTESIAN_POINT('Ctrl Pts',(-0.416738552178117,10.0260416666666,3.21171464055396));
#9360=CARTESIAN_POINT('Ctrl Pts',(0.427145446372979,9.91145833333345,3.23508431026218));
#9361=CARTESIAN_POINT('Ctrl Pts',(0.853764059103477,9.85416666666669,3.16284869617602));
#9362=CARTESIAN_POINT('Ctrl Pts',(1.65132730717562,9.73958333333332,2.85778233020993));
#9363=CARTESIAN_POINT('Ctrl Pts',(2.02194332446279,9.68229166666673,2.62503577071995));
#9364=CARTESIAN_POINT('Ctrl Pts',(2.64891940812677,9.56770833333328,2.03110939095704));
#9365=CARTESIAN_POINT('Ctrl Pts',(2.9050053877204,9.51041666666666,1.67013581324179));
#9366=CARTESIAN_POINT('Ctrl Pts',(3.26068667365192,9.39583333333334,0.872513118888943));
#9367=CARTESIAN_POINT('Ctrl Pts',(3.36010621991895,9.3385416666664,0.436162964680591));
#9368=CARTESIAN_POINT('Ctrl Pts',(3.38347588969759,9.22395833333361,-0.446569858875482));
#9369=CARTESIAN_POINT('Ctrl Pts',(3.30737803999626,9.16666666666689,-0.892605240889856));
#9370=CARTESIAN_POINT('Ctrl Pts',(2.98744487239941,9.05208333333312,-1.72606012326716));
#9371=CARTESIAN_POINT('Ctrl Pts',(2.74369959655829,8.99479166666641,-2.11313688270712));
#9372=CARTESIAN_POINT('Ctrl Pts',(2.1223029492484,8.8802083333336,-2.76758323401219));
#9373=CARTESIAN_POINT('Ctrl Pts',(1.74486862930228,8.82291666666647,-3.03466792985017));
#9374=CARTESIAN_POINT('Ctrl Pts',(0.911354300706321,8.70833333333354,-3.40521601753191));
#9375=CARTESIAN_POINT('Ctrl Pts',(0.455587377172263,8.6510416666665,-3.5084977992874));
#9376=CARTESIAN_POINT('Ctrl Pts',(-0.465994271367186,8.53645833333351,-3.53186746912954));
#9377=CARTESIAN_POINT('Ctrl Pts',(-0.93144642268745,8.47916666666683,-3.45190738381581));
#9378=CARTESIAN_POINT('Ctrl Pts',(-1.80079293934749,8.36458333333318,-3.11710741458959));
#9379=CARTESIAN_POINT('Ctrl Pts',(-2.20433044096071,8.30729166666683,-2.86236342239196));
#9380=CARTESIAN_POINT('Ctrl Pts',(-2.88624705988836,8.1927083333332,-2.21349650754444));
#9381=CARTESIAN_POINT('Ctrl Pts',(-3.1643304719878,8.13541666666656,-1.81960144535507));
#9382=CARTESIAN_POINT('Ctrl Pts',(-3.54974536140404,8.02083333333345,-0.950195482531384));
#9383=CARTESIAN_POINT('Ctrl Pts',(-3.65688937865929,7.96354166666637,-0.475011789653154));
#9384=CARTESIAN_POINT('Ctrl Pts',(-3.68025904855805,7.84895833333365,0.485418683848109));
#9385=CARTESIAN_POINT('Ctrl Pts',(-3.59643672763413,7.79166666666665,0.970287604495667));
#9386=CARTESIAN_POINT('Ctrl Pts',(-3.246769956781,7.67708333333337,1.8755257554172));
#9387=CARTESIAN_POINT('Ctrl Pts',(-2.98102724821984,7.61979166666659,2.29552399922486));
#9388=CARTESIAN_POINT('Ctrl Pts',(-2.30469006584627,7.50520833333343,3.00491088575395));
#9389=CARTESIAN_POINT('Ctrl Pts',(-1.89433426139971,7.44791666666668,3.29399301413121));
#9390=CARTESIAN_POINT('Ctrl Pts',(-0.989036664364609,7.33333333333333,3.69427470527038));
#9391=CARTESIAN_POINT('Ctrl Pts',(-0.49443620212397,7.27604166666629,3.80528095803426));
#9392=CARTESIAN_POINT('Ctrl Pts',(0.50484309631896,7.16145833333372,3.82865062798349));
#9393=CARTESIAN_POINT('Ctrl Pts',(1.00912878631411,7.10416666666678,3.74096607145172));
#9394=CARTESIAN_POINT('Ctrl Pts',(1.95025857147667,6.98958333333323,3.37643249897315));
#9395=CARTESIAN_POINT('Ctrl Pts',(2.38671755749636,6.93229166666724,3.09969107404422));
#9396=CARTESIAN_POINT('Ctrl Pts',(3.12357471161222,6.81770833333277,2.39588362415159));
#9397=CARTESIAN_POINT('Ctrl Pts',(3.42365555628099,6.76041666666712,1.96906707743673));
#9398=CARTESIAN_POINT('Ctrl Pts',(3.83880404913035,6.64583333333289,1.02787784620545));
#9399=CARTESIAN_POINT('Ctrl Pts',(3.95367253741186,6.58854166666688,0.51386061458762));
#9400=CARTESIAN_POINT('Ctrl Pts',(3.97704220740629,6.47395833333313,-0.524267508782646));
#9401=CARTESIAN_POINT('Ctrl Pts',(3.88549541526866,6.41666666666645,-1.04796996813959));
#9402=CARTESIAN_POINT('Ctrl Pts',(3.50609504116593,6.30208333333356,-2.02499138752914));
#9403=CARTESIAN_POINT('Ctrl Pts',(3.2183548998624,6.24479166666656,-2.47791111577681));
#9404=CARTESIAN_POINT('Ctrl Pts',(2.48707718246311,6.13020833333345,-3.24223853746153));
#9405=CARTESIAN_POINT('Ctrl Pts',(2.04379989346725,6.07291666666717,-3.55331809843599));
#9406=CARTESIAN_POINT('Ctrl Pts',(1.06671902805278,5.95833333333284,-3.9833333929851));
#9407=CARTESIAN_POINT('Ctrl Pts',(0.533285027040294,5.90104166666655,-4.10206411679133));
#9408=CARTESIAN_POINT('Ctrl Pts',(-0.543691921235359,5.78645833333346,-4.12543378682723));
#9409=CARTESIAN_POINT('Ctrl Pts',(-1.08681114997705,5.72916666666705,-4.03002475908303));
#9410=CARTESIAN_POINT('Ctrl Pts',(-2.0997242035696,5.61458333333296,-3.63575758336128));
#9411=CARTESIAN_POINT('Ctrl Pts',(-2.56910467406188,5.55729166666709,-3.33701872567955));
#9412=CARTESIAN_POINT('Ctrl Pts',(-3.36090236330622,5.44270833333292,-2.57827074077566));
#9413=CARTESIAN_POINT('Ctrl Pts',(-3.68298064059524,5.38541666666669,-2.11853270949184));
#9414=CARTESIAN_POINT('Ctrl Pts',(-4.12786273683561,5.27083333333332,-1.10556020990605));
#9415=CARTESIAN_POINT('Ctrl Pts',(-4.25045569617289,5.21354166666665,-0.552709439489368));
#9416=CARTESIAN_POINT('Ctrl Pts',(-4.27382536624608,5.09895833333335,0.563116333684488));
#9417=CARTESIAN_POINT('Ctrl Pts',(-4.17455410289751,5.04166666666663,1.12565233181968));
#9418=CARTESIAN_POINT('Ctrl Pts',(-3.76542012555652,4.92708333333338,2.17445701960491));
#9419=CARTESIAN_POINT('Ctrl Pts',(-3.45568255149002,4.86979166666659,2.66029823235588));
#9420=CARTESIAN_POINT('Ctrl Pts',(-2.6694642990949,4.75520833333342,3.47956618914197));
#9421=CARTESIAN_POINT('Ctrl Pts',(-2.19326552550957,4.69791666666658,3.81264318275876));
#9422=CARTESIAN_POINT('Ctrl Pts',(-1.14440139176617,4.58333333333343,4.27239208068185));
#9423=CARTESIAN_POINT('Ctrl Pts',(-0.572133851929879,4.52604166666658,4.39884727555618));
#9424=CARTESIAN_POINT('Ctrl Pts',(0.582540746125043,4.41145833333343,4.42221694566319));
#9425=CARTESIAN_POINT('Ctrl Pts',(1.16449351366757,4.35416666666679,4.31908344671154));
#9426=CARTESIAN_POINT('Ctrl Pts',(2.24918983563495,4.23958333333322,3.89508266775222));
#9427=CARTESIAN_POINT('Ctrl Pts',(2.75149179065353,4.18229166666676,3.57434637729919));
#9428=CARTESIAN_POINT('Ctrl Pts',(3.59823001497408,4.06770833333325,2.76065785741543));
#9429=CARTESIAN_POINT('Ctrl Pts',(3.94230572492611,4.01041666666671,2.26799834152485));
#9430=CARTESIAN_POINT('Ctrl Pts',(4.41692142452426,3.8958333333333,1.18324257362874));
#9431=CARTESIAN_POINT('Ctrl Pts',(4.54723885494094,3.83854166666642,0.591558264361257));
#9432=CARTESIAN_POINT('Ctrl Pts',(4.57060852507883,3.72395833333359,-0.601965158556466));
#9433=CARTESIAN_POINT('Ctrl Pts',(4.46361279052205,3.66666666666662,-1.20333469552689));
#9434=CARTESIAN_POINT('Ctrl Pts',(4.02474520995143,3.55208333333339,-2.32392265165357));
#9435=CARTESIAN_POINT('Ctrl Pts',(3.69301020310442,3.49479166666671,-2.84268534895739));
#9436=CARTESIAN_POINT('Ctrl Pts',(2.85185141573989,3.38020833333329,-3.71689384079999));
#9437=CARTESIAN_POINT('Ctrl Pts',(2.34273115753217,3.3229166666668,-4.07196826709743));
#9438=CARTESIAN_POINT('Ctrl Pts',(1.22208375549926,3.20833333333321,-4.56145076836271));
#9439=CARTESIAN_POINT('Ctrl Pts',(0.610982676792531,3.15104166666636,-4.6956304343271));
#9440=CARTESIAN_POINT('Ctrl Pts',(-0.621389570987771,3.03645833333365,-4.71900010449308));
#9441=CARTESIAN_POINT('Ctrl Pts',(-1.24217587738614,2.97916666666654,-4.60814213433379));
#9442=CARTESIAN_POINT('Ctrl Pts',(-2.39865546767225,2.86458333333347,-4.15440775214941));
#9443=CARTESIAN_POINT('Ctrl Pts',(-2.93387890726637,2.80729166666695,-3.81167402890586));
#9444=CARTESIAN_POINT('Ctrl Pts',(-3.83555766662078,2.69270833333305,-2.94304497406814));
#9445=CARTESIAN_POINT('Ctrl Pts',(-4.20163080927273,2.63541666666658,-2.41746397353493));
#9446=CARTESIAN_POINT('Ctrl Pts',(-4.70598011219716,2.52083333333343,-1.26092493737436));
#9447=CARTESIAN_POINT('Ctrl Pts',(-4.84402201371418,2.4635416666663,-0.630407089215845));
#9448=CARTESIAN_POINT('Ctrl Pts',(-4.86739168390641,2.34895833333371,0.64081398341115));
#9449=CARTESIAN_POINT('Ctrl Pts',(-4.75267147814405,2.29166666666676,1.28101705925391));
#9450=CARTESIAN_POINT('Ctrl Pts',(-4.28407029434887,2.17708333333325,2.47338828368244));
#9451=CARTESIAN_POINT('Ctrl Pts',(-3.93033785470491,2.11979166666664,3.0250724655795));
#9452=CARTESIAN_POINT('Ctrl Pts',(-3.0342385323988,2.00520833333337,3.95422149243741));
#9453=CARTESIAN_POINT('Ctrl Pts',(-2.49219678953305,1.94791666666658,4.33129335145034));
#9454=CARTESIAN_POINT('Ctrl Pts',(-1.29976611925407,1.83333333333343,4.85050945602931));
#9455=CARTESIAN_POINT('Ctrl Pts',(-0.6498315016342,1.77604166666627,4.99241359310244));
#9456=CARTESIAN_POINT('Ctrl Pts',(0.660238395829575,1.66145833333374,5.01578326331855));
#9457=CARTESIAN_POINT('Ctrl Pts',(1.31985824112059,1.60416666666663,4.89720082195578));
#9458=CARTESIAN_POINT('Ctrl Pts',(2.54812109969368,1.48958333333338,4.41373283654687));
#9459=CARTESIAN_POINT('Ctrl Pts',(3.1162660238978,1.43229166666683,4.04900168050008));
#9460=CARTESIAN_POINT('Ctrl Pts',(4.07288531824889,1.31770833333318,3.1254320907333));
#9461=CARTESIAN_POINT('Ctrl Pts',(4.460955893629,1.26041666666641,2.56692960553103));
#9462=CARTESIAN_POINT('Ctrl Pts',(4.99503879986042,1.1458333333336,1.33860730113391));
#9463=CARTESIAN_POINT('Ctrl Pts',(5.14080517249185,1.08854166666688,0.669255914044516));
#9464=CARTESIAN_POINT('Ctrl Pts',(5.16417484272955,0.973958333333134,-0.679662808239928));
#9465=CARTESIAN_POINT('Ctrl Pts',(5.04173016576313,0.916666666666909,-1.35869942299763));
#9466=CARTESIAN_POINT('Ctrl Pts',(4.54339537874923,0.8020833333331,-2.62285391569459));
#9467=CARTESIAN_POINT('Ctrl Pts',(4.16766550629842,0.744791666666392,-3.20745958221381));
#9468=CARTESIAN_POINT('Ctrl Pts',(3.21662564906467,0.630208333333619,-4.19154914406263));
#9469=CARTESIAN_POINT('Ctrl Pts',(2.6416624215197,0.572916666666411,-4.59061843581319));
#9470=CARTESIAN_POINT('Ctrl Pts',(1.3774484830231,0.4583333333336,-5.13956814368599));
#9471=CARTESIAN_POINT('Ctrl Pts',(0.688680326455284,0.401041666666677,-5.28919675188146));
#9472=CARTESIAN_POINT('Ctrl Pts',(-0.69908722065077,0.286458333333334,-5.31256642214034));
#9473=CARTESIAN_POINT('Ctrl Pts',(-1.39754060488348,0.229166666666838,-5.1862595095691));
#9474=CARTESIAN_POINT('Ctrl Pts',(-2.69758673168668,0.114583333333173,-4.67305792095299));
#9475=CARTESIAN_POINT('Ctrl Pts',(-3.29865313262765,0.0572916666665569,
-4.28632933922004));
#9476=CARTESIAN_POINT('Ctrl Pts',(-3.80443305520312,5.15793290147402E-15,
-3.79707426974638));
#9477=CARTESIAN_POINT('',(-4.04445221596811,5.20417042793042E-15,-4.05181100142375));
#9478=CARTESIAN_POINT('Origin',(-3.92444263558561,5.20417042793042E-15,
-3.92444263558507));
#9479=CARTESIAN_POINT('Ctrl Pts',(-2.3674783363584,10.9996616868026,-2.37117425835928));
#9480=CARTESIAN_POINT('Ctrl Pts',(-2.68598375393219,10.9424827912009,-2.07059921730022));
#9481=CARTESIAN_POINT('Ctrl Pts',(-2.94648697390286,10.8853038956006,-1.70515567693283));
#9482=CARTESIAN_POINT('Ctrl Pts',(-3.30964371429254,10.7708333333336,-0.896538039613314));
#9483=CARTESIAN_POINT('Ctrl Pts',(-3.41180604852602,10.7135416666669,-0.453515668913589));
#9484=CARTESIAN_POINT('Ctrl Pts',(-3.4379002366457,10.5989583333331,0.443108774718904));
#9485=CARTESIAN_POINT('Ctrl Pts',(-3.36178304590245,10.5416666666666,0.896358100460257));
#9486=CARTESIAN_POINT('Ctrl Pts',(-3.03905091217473,10.4270833333334,1.74368979436799));
#9487=CARTESIAN_POINT('Ctrl Pts',(-2.79252711081109,10.3697916666664,2.13742396723561));
#9488=CARTESIAN_POINT('Ctrl Pts',(-2.16323413009096,10.2552083333337,2.80361970275416));
#9489=CARTESIAN_POINT('Ctrl Pts',(-1.78068510549046,10.1979166666664,3.07579175088966));
#9490=CARTESIAN_POINT('Ctrl Pts',(-0.935379221363662,10.0833333333336,3.45417305821104));
#9491=CARTESIAN_POINT('Ctrl Pts',(-0.472940081479242,10.0260416666666,3.56019762788479));
#9492=CARTESIAN_POINT('Ctrl Pts',(0.462533187284589,9.91145833333345,3.58629181608734));
#9493=CARTESIAN_POINT('Ctrl Pts',(0.935199282188079,9.85416666666669,3.50631238974053));
#9494=CARTESIAN_POINT('Ctrl Pts',(1.81842261051809,9.73958333333332,3.16871345434639));
#9495=CARTESIAN_POINT('Ctrl Pts',(2.22861752543397,9.68229166666673,2.91119093668731));
#9496=CARTESIAN_POINT('Ctrl Pts',(2.92228352868554,9.56770833333328,2.25442768834444));
#9497=CARTESIAN_POINT('Ctrl Pts',(3.20545429299277,9.51041666666666,1.85541792160244));
#9498=CARTESIAN_POINT('Ctrl Pts',(3.59870240211769,9.39583333333334,0.974220403129539));
#9499=CARTESIAN_POINT('Ctrl Pts',(3.70858920724845,9.3385416666664,0.492364494026195));
#9500=CARTESIAN_POINT('Ctrl Pts',(3.73468339552408,9.22395833333361,-0.481957599831572));
#9501=CARTESIAN_POINT('Ctrl Pts',(3.65084173357628,9.16666666666689,-0.974040463933888));
#9502=CARTESIAN_POINT('Ctrl Pts',(3.29837599652037,9.05208333333312,-1.8931554266502));
#9503=CARTESIAN_POINT('Ctrl Pts',(3.02985476255422,8.99479166666641,-2.31981108364774));
#9504=CARTESIAN_POINT('Ctrl Pts',(2.34562124660724,8.8802083333336,-3.04094735460153));
#9505=CARTESIAN_POINT('Ctrl Pts',(1.93015073770027,8.82291666666647,-3.33511683510577));
#9506=CARTESIAN_POINT('Ctrl Pts',(1.01306158490958,8.70833333333354,-3.74323174601444));
#9507=CARTESIAN_POINT('Ctrl Pts',(0.511788906557484,8.6510416666665,-3.85698078661577));
#9508=CARTESIAN_POINT('Ctrl Pts',(-0.501382012362897,8.53645833333351,-3.88307497495716));
#9509=CARTESIAN_POINT('Ctrl Pts',(-1.01288164569554,8.47916666666683,-3.79537107740945));
#9510=CARTESIAN_POINT('Ctrl Pts',(-1.96788824276646,8.36458333333318,-3.42803853869692));
#9511=CARTESIAN_POINT('Ctrl Pts',(-2.41100464187403,8.30729166666683,-3.14851858841386));
#9512=CARTESIAN_POINT('Ctrl Pts',(-3.159611180505,8.1927083333332,-2.43681480487731));
#9513=CARTESIAN_POINT('Ctrl Pts',(-3.46477937722837,8.13541666666656,-2.00488355378617));
#9514=CARTESIAN_POINT('Ctrl Pts',(-3.8877610899016,8.02083333333345,-1.05190276670153));
#9515=CARTESIAN_POINT('Ctrl Pts',(-4.00537236598643,7.96354166666637,-0.531213319073915));
#9516=CARTESIAN_POINT('Ctrl Pts',(-4.03146655438691,7.84895833333365,0.520806424879362));
#9517=CARTESIAN_POINT('Ctrl Pts',(-3.93990042124014,7.79166666666665,1.05172282747159));
#9518=CARTESIAN_POINT('Ctrl Pts',(-3.55770108087595,7.67708333333337,2.04262105886835));
#9519=CARTESIAN_POINT('Ctrl Pts',(-3.26718241426475,7.61979166666659,2.50219820011361));
#9520=CARTESIAN_POINT('Ctrl Pts',(-2.52800836315612,7.50520833333343,3.27827500639517));
#9521=CARTESIAN_POINT('Ctrl Pts',(-2.07961636986072,7.44791666666668,3.59444191935829));
#9522=CARTESIAN_POINT('Ctrl Pts',(-1.09074394850484,7.33333333333333,4.03229043378143));
#9523=CARTESIAN_POINT('Ctrl Pts',(-0.550637731576509,7.27604166666629,4.15376394536062));
#9524=CARTESIAN_POINT('Ctrl Pts',(0.540230837381994,7.16145833333372,4.17985813381312));
#9525=CARTESIAN_POINT('Ctrl Pts',(1.09056400926098,7.10416666666678,4.08442976506864));
#9526=CARTESIAN_POINT('Ctrl Pts',(2.11735387495688,6.98958333333323,3.68736362305719));
#9527=CARTESIAN_POINT('Ctrl Pts',(2.59339175836345,6.93229166666724,3.38584624010982));
#9528=CARTESIAN_POINT('Ctrl Pts',(3.3969388322751,6.81770833333277,2.61920192144075));
#9529=CARTESIAN_POINT('Ctrl Pts',(3.72410446149635,6.76041666666712,2.15434918592434));
#9530=CARTESIAN_POINT('Ctrl Pts',(4.17681977765313,6.64583333333289,1.12958513031907));
#9531=CARTESIAN_POINT('Ctrl Pts',(4.30215552473732,6.58854166666688,0.570062144068889));
#9532=CARTESIAN_POINT('Ctrl Pts',(4.32824971323683,6.47395833333313,-0.559655249874413));
#9533=CARTESIAN_POINT('Ctrl Pts',(4.22895910889563,6.41666666666645,-1.12940519106012));
#9534=CARTESIAN_POINT('Ctrl Pts',(3.81702616523991,6.30208333333356,-2.19208669103568));
#9535=CARTESIAN_POINT('Ctrl Pts',(3.50451006594675,6.24479166666656,-2.68458531662391));
#9536=CARTESIAN_POINT('Ctrl Pts',(2.71039547973352,6.13020833333345,-3.51560265814439));
#9537=CARTESIAN_POINT('Ctrl Pts',(2.22908200197935,6.07291666666717,-3.85376700363998));
#9538=CARTESIAN_POINT('Ctrl Pts',(1.16842631214193,5.95833333333284,-4.32134912151925));
#9539=CARTESIAN_POINT('Ctrl Pts',(0.589486556547344,5.90104166666655,-4.45054710411593));
#9540=CARTESIAN_POINT('Ctrl Pts',(-0.579079662352908,5.78645833333346,-4.47664129265863));
#9541=CARTESIAN_POINT('Ctrl Pts',(-1.16824637287424,5.72916666666705,-4.37348845271886));
#9542=CARTESIAN_POINT('Ctrl Pts',(-2.26681950709949,5.61458333333296,-3.94668870742641));
#9543=CARTESIAN_POINT('Ctrl Pts',(-2.77577887489086,5.55729166666709,-3.62317389178086));
#9544=CARTESIAN_POINT('Ctrl Pts',(-3.6342664840072,5.44270833333292,-2.80158903802911));
#9545=CARTESIAN_POINT('Ctrl Pts',(-3.98342954578962,5.38541666666669,-2.30381481802579));
#9546=CARTESIAN_POINT('Ctrl Pts',(-4.46587846537937,5.27083333333332,-1.20726749397333));
#9547=CARTESIAN_POINT('Ctrl Pts',(-4.59893868349712,5.21354166666665,-0.608910969019916));
#9548=CARTESIAN_POINT('Ctrl Pts',(-4.62503287207784,5.09895833333335,0.598504074825539));
#9549=CARTESIAN_POINT('Ctrl Pts',(-4.51801779654147,5.04166666666663,1.20708755469526));
#9550=CARTESIAN_POINT('Ctrl Pts',(-4.07635124961353,4.92708333333338,2.34155232315641));
#9551=CARTESIAN_POINT('Ctrl Pts',(-3.74183771760646,4.86979166666659,2.86697243316876));
#9552=CARTESIAN_POINT('Ctrl Pts',(-2.89278259633321,4.75520833333342,3.75293030985906));
#9553=CARTESIAN_POINT('Ctrl Pts',(-2.37854763406351,4.69791666666658,4.1130920879442));
#9554=CARTESIAN_POINT('Ctrl Pts',(-1.24610867581347,4.58333333333343,4.61040780923455));
#9555=CARTESIAN_POINT('Ctrl Pts',(-0.628335381481812,4.52604166666658,4.74733026287932));
#9556=CARTESIAN_POINT('Ctrl Pts',(0.617928487287482,4.41145833333343,4.77342445149605));
#9557=CARTESIAN_POINT('Ctrl Pts',(1.24592873652376,4.35416666666679,4.66254714036264));
#9558=CARTESIAN_POINT('Ctrl Pts',(2.41628513920584,4.23958333333322,4.20601379180208));
#9559=CARTESIAN_POINT('Ctrl Pts',(2.95816599145146,4.18229166666676,3.86050154342994));
#9560=CARTESIAN_POINT('Ctrl Pts',(3.87159413570613,4.06770833333325,2.98397615463943));
#9561=CARTESIAN_POINT('Ctrl Pts',(4.24275463010319,4.01041666666671,2.45328045009706));
#9562=CARTESIAN_POINT('Ctrl Pts',(4.75493715308532,3.8958333333333,1.28494985765777));
#9563=CARTESIAN_POINT('Ctrl Pts',(4.89572184226387,3.83854166666642,0.647759793932574));
#9564=CARTESIAN_POINT('Ctrl Pts',(4.9218160309119,3.72395833333359,-0.637352899738291));
#9565=CARTESIAN_POINT('Ctrl Pts',(4.80707648417982,3.66666666666662,-1.28476991836542));
#9566=CARTESIAN_POINT('Ctrl Pts',(4.33567633399462,3.55208333333339,-2.49101795524214));
#9567=CARTESIAN_POINT('Ctrl Pts',(3.97916536924807,3.49479166666671,-3.04935954974168));
#9568=CARTESIAN_POINT('Ctrl Pts',(3.075169712951,3.38020833333329,-3.99025796154567));
#9569=CARTESIAN_POINT('Ctrl Pts',(2.52801326612096,3.3229166666668,-4.37241717226731));
#9570=CARTESIAN_POINT('Ctrl Pts',(1.3237910395117,3.20833333333321,-4.89946649693097));
#9571=CARTESIAN_POINT('Ctrl Pts',(0.667184206381905,3.15104166666636,-5.04411342164931));
#9572=CARTESIAN_POINT('Ctrl Pts',(-0.656777312187654,3.03645833333365,-5.07020761032686));
#9573=CARTESIAN_POINT('Ctrl Pts',(-1.32361110020785,2.97916666666654,-4.95160582799841));
#9574=CARTESIAN_POINT('Ctrl Pts',(-2.56575077127763,2.86458333333347,-4.46533887618575));
#9575=CARTESIAN_POINT('Ctrl Pts',(-3.1405531080382,2.80729166666695,-4.09782919506089));
#9576=CARTESIAN_POINT('Ctrl Pts',(-4.10892178737893,2.69270833333305,-3.16636327126786));
#9577=CARTESIAN_POINT('Ctrl Pts',(-4.50207971443576,2.63541666666658,-2.60274608213879));
#9578=CARTESIAN_POINT('Ctrl Pts',(-5.04399584077227,2.52083333333343,-1.36263222137173));
#9579=CARTESIAN_POINT('Ctrl Pts',(-5.1925050010359,2.4635416666663,-0.686608618821642));
#9580=CARTESIAN_POINT('Ctrl Pts',(-5.21859918974068,2.34895833333371,0.67620172462746));
#9581=CARTESIAN_POINT('Ctrl Pts',(-5.09613517181383,2.29166666666676,1.36245228206106));
#9582=CARTESIAN_POINT('Ctrl Pts',(-4.59500141838005,2.17708333333325,2.64048358730238));
#9583=CARTESIAN_POINT('Ctrl Pts',(-4.21649302087059,2.11979166666664,3.23174666634004));
#9584=CARTESIAN_POINT('Ctrl Pts',(-3.25755682958786,2.00520833333337,4.22758561320685));
#9585=CARTESIAN_POINT('Ctrl Pts',(-2.67747889815098,1.94791666666658,4.63174225660692));
#9586=CARTESIAN_POINT('Ctrl Pts',(-1.40147340323737,1.83333333333343,5.18852518461089));
#9587=CARTESIAN_POINT('Ctrl Pts',(-0.706033031254986,1.77604166666627,5.34089658042353));
#9588=CARTESIAN_POINT('Ctrl Pts',(0.695626137060878,1.66145833333374,5.36699076915345));
#9589=CARTESIAN_POINT('Ctrl Pts',(1.40129346391331,1.60416666666663,5.24066451563091));
#9590=CARTESIAN_POINT('Ctrl Pts',(2.71521640332806,1.48958333333338,4.7246639605727));
#9591=CARTESIAN_POINT('Ctrl Pts',(3.32294022464786,1.43229166666683,4.33515684667557));
#9592=CARTESIAN_POINT('Ctrl Pts',(4.34624943902881,1.31770833333318,3.34875038791256));
#9593=CARTESIAN_POINT('Ctrl Pts',(4.76140479878007,1.26041666666641,2.75221171416214));
#9594=CARTESIAN_POINT('Ctrl Pts',(5.3330545284475,1.1458333333336,1.44031458510402));
#9595=CARTESIAN_POINT('Ctrl Pts',(5.48928815981245,1.08854166666688,0.72545744367903));
#9596=CARTESIAN_POINT('Ctrl Pts',(5.51538234856494,0.973958333333134,-0.715050549484959));
#9597=CARTESIAN_POINT('Ctrl Pts',(5.38519385944284,0.916666666666909,-1.44013464577813));
#9598=CARTESIAN_POINT('Ctrl Pts',(4.85432650277048,0.8020833333331,-2.7899492193412));
#9599=CARTESIAN_POINT('Ctrl Pts',(4.4538206724838,0.744791666666392,-3.4141337829535));
#9600=CARTESIAN_POINT('Ctrl Pts',(3.43994394623404,0.630208333333619,-4.46491326485293));
#9601=CARTESIAN_POINT('Ctrl Pts',(2.82694453016243,0.572916666666411,-4.89106734095877));
#9602=CARTESIAN_POINT('Ctrl Pts',(1.47915576698159,0.4583333333336,-5.47758387227856));
#9603=CARTESIAN_POINT('Ctrl Pts',(0.744881856102772,0.401041666666677,-5.63767973920226));
#9604=CARTESIAN_POINT('Ctrl Pts',(-0.73447496190878,0.286458333333334,-5.66377392797554));
#9605=CARTESIAN_POINT('Ctrl Pts',(-1.4789758276525,0.229166666666838,-5.52972320325324));
#9606=CARTESIAN_POINT('Ctrl Pts',(-2.86468203534475,0.114583333333173,-4.9839890449698));
#9607=CARTESIAN_POINT('Ctrl Pts',(-3.50532733285514,0.0572916666665569,
-4.5724845058884));
#9608=CARTESIAN_POINT('Ctrl Pts',(-4.04445221596811,5.20417042793042E-15,
-4.05181100142375));
#9609=CARTESIAN_POINT('Ctrl Pts',(-2.36559314293001,11.,-2.37295192838617));
#9610=CARTESIAN_POINT('Ctrl Pts',(-2.68495589138643,10.9427083333325,-2.0720405595763));
#9611=CARTESIAN_POINT('Ctrl Pts',(-2.94612920879841,10.8854166666664,-1.70595228936294));
#9612=CARTESIAN_POINT('Ctrl Pts',(-3.30964371429254,10.7708333333336,-0.896538039613314));
#9613=CARTESIAN_POINT('Ctrl Pts',(-3.41180604852602,10.7135416666669,-0.453515668913589));
#9614=CARTESIAN_POINT('Ctrl Pts',(-3.4379002366457,10.5989583333331,0.443108774718904));
#9615=CARTESIAN_POINT('Ctrl Pts',(-3.36178304590245,10.5416666666666,0.896358100460257));
#9616=CARTESIAN_POINT('Ctrl Pts',(-3.03905091217473,10.4270833333334,1.74368979436799));
#9617=CARTESIAN_POINT('Ctrl Pts',(-2.79252711081109,10.3697916666664,2.13742396723561));
#9618=CARTESIAN_POINT('Ctrl Pts',(-2.16323413009096,10.2552083333337,2.80361970275416));
#9619=CARTESIAN_POINT('Ctrl Pts',(-1.78068510549046,10.1979166666664,3.07579175088966));
#9620=CARTESIAN_POINT('Ctrl Pts',(-0.935379221363662,10.0833333333336,3.45417305821104));
#9621=CARTESIAN_POINT('Ctrl Pts',(-0.472940081479242,10.0260416666666,3.56019762788479));
#9622=CARTESIAN_POINT('Ctrl Pts',(0.462533187284589,9.91145833333345,3.58629181608734));
#9623=CARTESIAN_POINT('Ctrl Pts',(0.935199282188079,9.85416666666669,3.50631238974053));
#9624=CARTESIAN_POINT('Ctrl Pts',(1.81842261051809,9.73958333333332,3.16871345434639));
#9625=CARTESIAN_POINT('Ctrl Pts',(2.22861752543397,9.68229166666673,2.91119093668731));
#9626=CARTESIAN_POINT('Ctrl Pts',(2.92228352868554,9.56770833333328,2.25442768834444));
#9627=CARTESIAN_POINT('Ctrl Pts',(3.20545429299277,9.51041666666666,1.85541792160244));
#9628=CARTESIAN_POINT('Ctrl Pts',(3.59870240211769,9.39583333333334,0.974220403129539));
#9629=CARTESIAN_POINT('Ctrl Pts',(3.70858920724845,9.3385416666664,0.492364494026195));
#9630=CARTESIAN_POINT('Ctrl Pts',(3.73468339552408,9.22395833333361,-0.481957599831572));
#9631=CARTESIAN_POINT('Ctrl Pts',(3.65084173357628,9.16666666666689,-0.974040463933888));
#9632=CARTESIAN_POINT('Ctrl Pts',(3.29837599652037,9.05208333333312,-1.8931554266502));
#9633=CARTESIAN_POINT('Ctrl Pts',(3.02985476255422,8.99479166666641,-2.31981108364774));
#9634=CARTESIAN_POINT('Ctrl Pts',(2.34562124660724,8.8802083333336,-3.04094735460153));
#9635=CARTESIAN_POINT('Ctrl Pts',(1.93015073770027,8.82291666666647,-3.33511683510577));
#9636=CARTESIAN_POINT('Ctrl Pts',(1.01306158490958,8.70833333333354,-3.74323174601444));
#9637=CARTESIAN_POINT('Ctrl Pts',(0.511788906557484,8.6510416666665,-3.85698078661577));
#9638=CARTESIAN_POINT('Ctrl Pts',(-0.501382012362897,8.53645833333351,-3.88307497495716));
#9639=CARTESIAN_POINT('Ctrl Pts',(-1.01288164569554,8.47916666666683,-3.79537107740945));
#9640=CARTESIAN_POINT('Ctrl Pts',(-1.96788824276646,8.36458333333318,-3.42803853869692));
#9641=CARTESIAN_POINT('Ctrl Pts',(-2.41100464187403,8.30729166666683,-3.14851858841386));
#9642=CARTESIAN_POINT('Ctrl Pts',(-3.159611180505,8.1927083333332,-2.43681480487731));
#9643=CARTESIAN_POINT('Ctrl Pts',(-3.46477937722837,8.13541666666656,-2.00488355378617));
#9644=CARTESIAN_POINT('Ctrl Pts',(-3.8877610899016,8.02083333333345,-1.05190276670153));
#9645=CARTESIAN_POINT('Ctrl Pts',(-4.00537236598643,7.96354166666637,-0.531213319073915));
#9646=CARTESIAN_POINT('Ctrl Pts',(-4.03146655438691,7.84895833333365,0.520806424879362));
#9647=CARTESIAN_POINT('Ctrl Pts',(-3.93990042124014,7.79166666666665,1.05172282747159));
#9648=CARTESIAN_POINT('Ctrl Pts',(-3.55770108087595,7.67708333333337,2.04262105886835));
#9649=CARTESIAN_POINT('Ctrl Pts',(-3.26718241426475,7.61979166666659,2.50219820011361));
#9650=CARTESIAN_POINT('Ctrl Pts',(-2.52800836315612,7.50520833333343,3.27827500639517));
#9651=CARTESIAN_POINT('Ctrl Pts',(-2.07961636986072,7.44791666666668,3.59444191935829));
#9652=CARTESIAN_POINT('Ctrl Pts',(-1.09074394850484,7.33333333333333,4.03229043378143));
#9653=CARTESIAN_POINT('Ctrl Pts',(-0.550637731576509,7.27604166666629,4.15376394536062));
#9654=CARTESIAN_POINT('Ctrl Pts',(0.540230837381994,7.16145833333372,4.17985813381312));
#9655=CARTESIAN_POINT('Ctrl Pts',(1.09056400926098,7.10416666666678,4.08442976506864));
#9656=CARTESIAN_POINT('Ctrl Pts',(2.11735387495688,6.98958333333323,3.68736362305719));
#9657=CARTESIAN_POINT('Ctrl Pts',(2.59339175836345,6.93229166666724,3.38584624010982));
#9658=CARTESIAN_POINT('Ctrl Pts',(3.3969388322751,6.81770833333277,2.61920192144075));
#9659=CARTESIAN_POINT('Ctrl Pts',(3.72410446149635,6.76041666666712,2.15434918592434));
#9660=CARTESIAN_POINT('Ctrl Pts',(4.17681977765313,6.64583333333289,1.12958513031907));
#9661=CARTESIAN_POINT('Ctrl Pts',(4.30215552473732,6.58854166666688,0.570062144068889));
#9662=CARTESIAN_POINT('Ctrl Pts',(4.32824971323683,6.47395833333313,-0.559655249874413));
#9663=CARTESIAN_POINT('Ctrl Pts',(4.22895910889563,6.41666666666645,-1.12940519106012));
#9664=CARTESIAN_POINT('Ctrl Pts',(3.81702616523991,6.30208333333356,-2.19208669103568));
#9665=CARTESIAN_POINT('Ctrl Pts',(3.50451006594675,6.24479166666656,-2.68458531662391));
#9666=CARTESIAN_POINT('Ctrl Pts',(2.71039547973352,6.13020833333345,-3.51560265814439));
#9667=CARTESIAN_POINT('Ctrl Pts',(2.22908200197935,6.07291666666717,-3.85376700363998));
#9668=CARTESIAN_POINT('Ctrl Pts',(1.16842631214193,5.95833333333284,-4.32134912151925));
#9669=CARTESIAN_POINT('Ctrl Pts',(0.589486556547344,5.90104166666655,-4.45054710411593));
#9670=CARTESIAN_POINT('Ctrl Pts',(-0.579079662352908,5.78645833333346,-4.47664129265863));
#9671=CARTESIAN_POINT('Ctrl Pts',(-1.16824637287424,5.72916666666705,-4.37348845271886));
#9672=CARTESIAN_POINT('Ctrl Pts',(-2.26681950709949,5.61458333333296,-3.94668870742641));
#9673=CARTESIAN_POINT('Ctrl Pts',(-2.77577887489086,5.55729166666709,-3.62317389178086));
#9674=CARTESIAN_POINT('Ctrl Pts',(-3.6342664840072,5.44270833333292,-2.80158903802911));
#9675=CARTESIAN_POINT('Ctrl Pts',(-3.98342954578962,5.38541666666669,-2.30381481802579));
#9676=CARTESIAN_POINT('Ctrl Pts',(-4.46587846537937,5.27083333333332,-1.20726749397333));
#9677=CARTESIAN_POINT('Ctrl Pts',(-4.59893868349712,5.21354166666665,-0.608910969019916));
#9678=CARTESIAN_POINT('Ctrl Pts',(-4.62503287207784,5.09895833333335,0.598504074825539));
#9679=CARTESIAN_POINT('Ctrl Pts',(-4.51801779654147,5.04166666666663,1.20708755469526));
#9680=CARTESIAN_POINT('Ctrl Pts',(-4.07635124961353,4.92708333333338,2.34155232315641));
#9681=CARTESIAN_POINT('Ctrl Pts',(-3.74183771760646,4.86979166666659,2.86697243316876));
#9682=CARTESIAN_POINT('Ctrl Pts',(-2.89278259633321,4.75520833333342,3.75293030985906));
#9683=CARTESIAN_POINT('Ctrl Pts',(-2.37854763406351,4.69791666666658,4.1130920879442));
#9684=CARTESIAN_POINT('Ctrl Pts',(-1.24610867581347,4.58333333333343,4.61040780923455));
#9685=CARTESIAN_POINT('Ctrl Pts',(-0.628335381481812,4.52604166666658,4.74733026287932));
#9686=CARTESIAN_POINT('Ctrl Pts',(0.617928487287482,4.41145833333343,4.77342445149605));
#9687=CARTESIAN_POINT('Ctrl Pts',(1.24592873652376,4.35416666666679,4.66254714036264));
#9688=CARTESIAN_POINT('Ctrl Pts',(2.41628513920584,4.23958333333322,4.20601379180208));
#9689=CARTESIAN_POINT('Ctrl Pts',(2.95816599145146,4.18229166666676,3.86050154342994));
#9690=CARTESIAN_POINT('Ctrl Pts',(3.87159413570613,4.06770833333325,2.98397615463943));
#9691=CARTESIAN_POINT('Ctrl Pts',(4.24275463010319,4.01041666666671,2.45328045009706));
#9692=CARTESIAN_POINT('Ctrl Pts',(4.75493715308532,3.8958333333333,1.28494985765777));
#9693=CARTESIAN_POINT('Ctrl Pts',(4.89572184226387,3.83854166666642,0.647759793932574));
#9694=CARTESIAN_POINT('Ctrl Pts',(4.9218160309119,3.72395833333359,-0.637352899738291));
#9695=CARTESIAN_POINT('Ctrl Pts',(4.80707648417982,3.66666666666662,-1.28476991836542));
#9696=CARTESIAN_POINT('Ctrl Pts',(4.33567633399462,3.55208333333339,-2.49101795524214));
#9697=CARTESIAN_POINT('Ctrl Pts',(3.97916536924807,3.49479166666671,-3.04935954974168));
#9698=CARTESIAN_POINT('Ctrl Pts',(3.075169712951,3.38020833333329,-3.99025796154567));
#9699=CARTESIAN_POINT('Ctrl Pts',(2.52801326612096,3.3229166666668,-4.37241717226731));
#9700=CARTESIAN_POINT('Ctrl Pts',(1.3237910395117,3.20833333333321,-4.89946649693097));
#9701=CARTESIAN_POINT('Ctrl Pts',(0.667184206381905,3.15104166666636,-5.04411342164931));
#9702=CARTESIAN_POINT('Ctrl Pts',(-0.656777312187654,3.03645833333365,-5.07020761032686));
#9703=CARTESIAN_POINT('Ctrl Pts',(-1.32361110020785,2.97916666666654,-4.95160582799841));
#9704=CARTESIAN_POINT('Ctrl Pts',(-2.56575077127763,2.86458333333347,-4.46533887618575));
#9705=CARTESIAN_POINT('Ctrl Pts',(-3.1405531080382,2.80729166666695,-4.09782919506089));
#9706=CARTESIAN_POINT('Ctrl Pts',(-4.10892178737893,2.69270833333305,-3.16636327126786));
#9707=CARTESIAN_POINT('Ctrl Pts',(-4.50207971443576,2.63541666666658,-2.60274608213879));
#9708=CARTESIAN_POINT('Ctrl Pts',(-5.04399584077227,2.52083333333343,-1.36263222137173));
#9709=CARTESIAN_POINT('Ctrl Pts',(-5.1925050010359,2.4635416666663,-0.686608618821642));
#9710=CARTESIAN_POINT('Ctrl Pts',(-5.21859918974068,2.34895833333371,0.67620172462746));
#9711=CARTESIAN_POINT('Ctrl Pts',(-5.09613517181383,2.29166666666676,1.36245228206106));
#9712=CARTESIAN_POINT('Ctrl Pts',(-4.59500141838005,2.17708333333325,2.64048358730238));
#9713=CARTESIAN_POINT('Ctrl Pts',(-4.21649302087059,2.11979166666664,3.23174666634004));
#9714=CARTESIAN_POINT('Ctrl Pts',(-3.25755682958786,2.00520833333337,4.22758561320685));
#9715=CARTESIAN_POINT('Ctrl Pts',(-2.67747889815098,1.94791666666658,4.63174225660692));
#9716=CARTESIAN_POINT('Ctrl Pts',(-1.40147340323737,1.83333333333343,5.18852518461089));
#9717=CARTESIAN_POINT('Ctrl Pts',(-0.706033031254986,1.77604166666627,5.34089658042353));
#9718=CARTESIAN_POINT('Ctrl Pts',(0.695626137060878,1.66145833333374,5.36699076915345));
#9719=CARTESIAN_POINT('Ctrl Pts',(1.40129346391331,1.60416666666663,5.24066451563091));
#9720=CARTESIAN_POINT('Ctrl Pts',(2.71521640332806,1.48958333333338,4.7246639605727));
#9721=CARTESIAN_POINT('Ctrl Pts',(3.32294022464786,1.43229166666683,4.33515684667557));
#9722=CARTESIAN_POINT('Ctrl Pts',(4.34624943902881,1.31770833333318,3.34875038791256));
#9723=CARTESIAN_POINT('Ctrl Pts',(4.76140479878007,1.26041666666641,2.75221171416214));
#9724=CARTESIAN_POINT('Ctrl Pts',(5.3330545284475,1.1458333333336,1.44031458510402));
#9725=CARTESIAN_POINT('Ctrl Pts',(5.48928815981245,1.08854166666688,0.72545744367903));
#9726=CARTESIAN_POINT('Ctrl Pts',(5.51538234856494,0.973958333333134,-0.715050549484959));
#9727=CARTESIAN_POINT('Ctrl Pts',(5.38519385944284,0.916666666666909,-1.44013464577813));
#9728=CARTESIAN_POINT('Ctrl Pts',(4.85432650277048,0.8020833333331,-2.7899492193412));
#9729=CARTESIAN_POINT('Ctrl Pts',(4.4538206724838,0.744791666666392,-3.4141337829535));
#9730=CARTESIAN_POINT('Ctrl Pts',(3.43994394623404,0.630208333333619,-4.46491326485293));
#9731=CARTESIAN_POINT('Ctrl Pts',(2.82694453016243,0.572916666666411,-4.89106734095877));
#9732=CARTESIAN_POINT('Ctrl Pts',(1.47915576698159,0.4583333333336,-5.47758387227856));
#9733=CARTESIAN_POINT('Ctrl Pts',(0.744881856102772,0.401041666666677,-5.63767973920226));
#9734=CARTESIAN_POINT('Ctrl Pts',(-0.73447496190878,0.286458333333334,-5.66377392797554));
#9735=CARTESIAN_POINT('Ctrl Pts',(-1.4789758276525,0.229166666666838,-5.52972320325324));
#9736=CARTESIAN_POINT('Ctrl Pts',(-2.86468203534475,0.114583333333173,-4.9839890449698));
#9737=CARTESIAN_POINT('Ctrl Pts',(-3.50532733285514,0.0572916666665569,
-4.5724845058884));
#9738=CARTESIAN_POINT('Ctrl Pts',(-4.04445221596811,5.20417042793042E-15,
-4.05181100142375));
#9739=CARTESIAN_POINT('Ctrl Pts',(-2.40035683308082,11.3467255152722,-2.34019673175572));
#9740=CARTESIAN_POINT('Ctrl Pts',(-2.71543193620083,11.2894338486048,-2.03473480641482));
#9741=CARTESIAN_POINT('Ctrl Pts',(-2.97141448964516,11.2321421819387,-1.66495030044034));
#9742=CARTESIAN_POINT('Ctrl Pts',(-3.32352361490692,11.1175588486058,-0.850409340498224));
#9743=CARTESIAN_POINT('Ctrl Pts',(-3.4194758201212,11.0602671819391,-0.405958512493029));
#9744=CARTESIAN_POINT('Ctrl Pts',(-3.43307090382695,10.9456838486053,0.491037743700738));
#9745=CARTESIAN_POINT('Ctrl Pts',(-3.35066965504748,10.8883921819389,0.943230278421825));
#9746=CARTESIAN_POINT('Ctrl Pts',(-3.01624756806638,10.7738088486056,1.78612228216488));
#9747=CARTESIAN_POINT('Ctrl Pts',(-2.76432247051982,10.7165171819386,2.17647530254211));
#9748=CARTESIAN_POINT('Ctrl Pts',(-2.12592837712132,10.6019338486059,2.83409574774927));
#9749=CARTESIAN_POINT('Ctrl Pts',(-1.7396831165707,10.5446421819387,3.10107703174287));
#9750=CARTESIAN_POINT('Ctrl Pts',(-0.889250522245734,10.4300588486058,3.46805295881896));
#9751=CARTESIAN_POINT('Ctrl Pts',(-0.425382925058827,10.3727671819388,3.56786739948684));
#9752=CARTESIAN_POINT('Ctrl Pts',(0.510462156266568,10.2581838486057,3.58146248326171));
#9753=CARTESIAN_POINT('Ctrl Pts',(0.982071460151994,10.2008921819389,3.49519899889172));
#9754=CARTESIAN_POINT('Ctrl Pts',(1.86085509831263,10.0863088486056,3.14591011023186));
#9755=CARTESIAN_POINT('Ctrl Pts',(2.26766886074488,10.029017181939,2.88298629640079));
#9756=CARTESIAN_POINT('Ctrl Pts',(2.95275957367625,9.91443384860552,2.21712193537007));
#9757=CARTESIAN_POINT('Ctrl Pts',(3.2307395738517,9.8571421819389,1.81441593268519));
#9758=CARTESIAN_POINT('Ctrl Pts',(3.61258230271989,9.74255884860558,0.9280917040091));
#9759=CARTESIAN_POINT('Ctrl Pts',(3.71625897885657,9.68526718193864,0.444807337606009));
#9760=CARTESIAN_POINT('Ctrl Pts',(3.72985406269238,9.57068384860584,-0.52988656881378));
#9761=CARTESIAN_POINT('Ctrl Pts',(3.63972834273301,9.51339218193913,-1.02091264189992));
#9762=CARTESIAN_POINT('Ctrl Pts',(3.2755726524003,9.39880884860535,-1.93558791444263));
#9763=CARTESIAN_POINT('Ctrl Pts',(3.00165012227183,9.34151718193865,-2.35886241896257));
#9764=CARTESIAN_POINT('Ctrl Pts',(2.30831549362873,9.22693384860583,-3.07142339958832));
#9765=CARTESIAN_POINT('Ctrl Pts',(1.88914874878537,9.1696421819387,-3.3604021159697));
#9766=CARTESIAN_POINT('Ctrl Pts',(0.966932885786784,9.05505884860578,-3.75711164661164));
#9767=CARTESIAN_POINT('Ctrl Pts',(0.46423175013744,8.99776718193874,-3.86465055822944));
#9768=CARTESIAN_POINT('Ctrl Pts',(-0.549310981345247,8.88318384860575,-3.87824564211992));
#9769=CARTESIAN_POINT('Ctrl Pts',(-1.05975382366345,8.82589218193907,-3.78425768657106));
#9770=CARTESIAN_POINT('Ctrl Pts',(-2.01032073055702,8.71130884860541,-3.40523519457197));
#9771=CARTESIAN_POINT('Ctrl Pts',(-2.45005597719243,8.65401718193906,-3.12031394813519));
#9772=CARTESIAN_POINT('Ctrl Pts',(-3.19008722548821,8.53943384860543,-2.39950905189507));
#9773=CARTESIAN_POINT('Ctrl Pts',(-3.49006465809683,8.48214218193879,-1.96388156487328));
#9774=CARTESIAN_POINT('Ctrl Pts',(-3.90164099049427,8.36755884860569,-1.00577406757672));
#9775=CARTESIAN_POINT('Ctrl Pts',(-4.01304213760465,8.3102671819386,-0.483656162654029));
#9776=CARTESIAN_POINT('Ctrl Pts',(-4.02663722154512,8.19568384860588,0.568735393861871));
#9777=CARTESIAN_POINT('Ctrl Pts',(-3.92878703040616,8.13839218193865,1.09859500544122));
#9778=CARTESIAN_POINT('Ctrl Pts',(-3.5348977367466,8.02380884860583,2.08505354665718));
#9779=CARTESIAN_POINT('Ctrl Pts',(-3.23897777398945,7.96651718193906,2.54124953543508));
#9780=CARTESIAN_POINT('Ctrl Pts',(-2.49070261017052,7.85193384860543,3.30875105137532));
#9781=CARTESIAN_POINT('Ctrl Pts',(-2.03861438094966,7.79464218193892,3.61972720023077));
#9782=CARTESIAN_POINT('Ctrl Pts',(-1.0446152493782,7.68005884860556,4.04617033437007));
#9783=CARTESIAN_POINT('Ctrl Pts',(-0.503080575156725,7.62276718193853,4.16143371698328));
#9784=CARTESIAN_POINT('Ctrl Pts',(0.588159806364604,7.50818384860596,4.17502880096689));
#9785=CARTESIAN_POINT('Ctrl Pts',(1.13743618723204,7.45089218193902,4.07331637423875));
#9786=CARTESIAN_POINT('Ctrl Pts',(2.15978636274428,7.33630884860546,3.66456027892374));
#9787=CARTESIAN_POINT('Ctrl Pts',(2.63244309368768,7.27901718193947,3.35764159983753));
#9788=CARTESIAN_POINT('Ctrl Pts',(3.42741487725249,7.16443384860501,2.58189616845213));
#9789=CARTESIAN_POINT('Ctrl Pts',(3.74938974237272,7.10714218193936,2.11334719701498));
#9790=CARTESIAN_POINT('Ctrl Pts',(4.19069967823789,6.99255884860513,1.08345643119075));
#9791=CARTESIAN_POINT('Ctrl Pts',(4.30982529636403,6.93526718193912,0.522504987649244));
#9792=CARTESIAN_POINT('Ctrl Pts',(4.32342038038655,6.82068384860537,-0.607584218857162));
#9793=CARTESIAN_POINT('Ctrl Pts',(4.21784571806929,6.76339218193869,-1.17627736903264));
#9794=CARTESIAN_POINT('Ctrl Pts',(3.79422282110293,6.6488088486058,-2.23451917882162));
#9795=CARTESIAN_POINT('Ctrl Pts',(3.47630542567715,6.5915171819388,-2.72363665195073));
#9796=CARTESIAN_POINT('Ctrl Pts',(2.67308972674222,6.47693384860569,-3.54607870311919));
#9797=CARTESIAN_POINT('Ctrl Pts',(2.18808001307138,6.41964218193941,-3.87905228451955));
#9798=CARTESIAN_POINT('Ctrl Pts',(1.1222976130122,6.30505884860508,-4.33522902210081));
#9799=CARTESIAN_POINT('Ctrl Pts',(0.541929400127819,6.24776718193879,-4.45821687574607));
#9800=CARTESIAN_POINT('Ctrl Pts',(-0.627008631335778,6.1331838486057,-4.47181195980492));
#9801=CARTESIAN_POINT('Ctrl Pts',(-1.21511855084784,6.07589218193929,-4.3623750618956));
#9802=CARTESIAN_POINT('Ctrl Pts',(-2.30925199488436,5.9613088486052,-3.92388536328634));
#9803=CARTESIAN_POINT('Ctrl Pts',(-2.81483021022013,5.90401718193932,-3.59496925151373));
#9804=CARTESIAN_POINT('Ctrl Pts',(-3.66474252897955,5.78943384860516,-2.76428328503534));
#9805=CARTESIAN_POINT('Ctrl Pts',(-4.0087148266721,5.73214218193892,-2.26281282911923));
#9806=CARTESIAN_POINT('Ctrl Pts',(-4.47975836595802,5.61755884860556,-1.1611387948422));
#9807=CARTESIAN_POINT('Ctrl Pts',(-4.60660845513052,5.56026718193889,-0.561353812600464));
#9808=CARTESIAN_POINT('Ctrl Pts',(-4.62020353922087,5.44568384860559,0.646433043808482));
#9809=CARTESIAN_POINT('Ctrl Pts',(-4.50690440572112,5.38839218193887,1.25395973267003));
#9810=CARTESIAN_POINT('Ctrl Pts',(-4.05354790547054,5.27380884860562,2.38398481094011));
#9811=CARTESIAN_POINT('Ctrl Pts',(-3.71363307734148,5.21651718193883,2.90602376850005));
#9812=CARTESIAN_POINT('Ctrl Pts',(-2.85547684333729,5.10193384860566,3.78340635482939));
#9813=CARTESIAN_POINT('Ctrl Pts',(-2.33754564515818,5.04464218193881,4.13837736882935));
#9814=CARTESIAN_POINT('Ctrl Pts',(-1.1999799766811,4.93005884860567,4.62428770981052));
#9815=CARTESIAN_POINT('Ctrl Pts',(-0.580778225062417,4.87276718193882,4.75500003451575));
#9816=CARTESIAN_POINT('Ctrl Pts',(0.665857456270481,4.75818384860566,4.76859511863605));
#9817=CARTESIAN_POINT('Ctrl Pts',(1.2928009144995,4.70089218193903,4.65143374954513));
#9818=CARTESIAN_POINT('Ctrl Pts',(2.45871762698856,4.58630884860546,4.18321044765625));
#9819=CARTESIAN_POINT('Ctrl Pts',(2.99721732678471,4.529017181939,3.83229690316695));
#9820=CARTESIAN_POINT('Ctrl Pts',(3.9020701806745,4.41443384860549,2.94667040164152));
#9821=CARTESIAN_POINT('Ctrl Pts',(4.2680399109909,4.35714218193895,2.41227846119283));
#9822=CARTESIAN_POINT('Ctrl Pts',(4.76881705365873,4.24255884860554,1.2388211585243));
#9823=CARTESIAN_POINT('Ctrl Pts',(4.90339161390277,4.18526718193866,0.600202637513305));
#9824=CARTESIAN_POINT('Ctrl Pts',(4.91698669804943,4.07068384860583,-0.685281868721417));
#9825=CARTESIAN_POINT('Ctrl Pts',(4.79596309336461,4.01339218193886,-1.33164209634213));
#9826=CARTESIAN_POINT('Ctrl Pts',(4.31287298984649,3.89880884860562,-2.53345044302389));
#9827=CARTESIAN_POINT('Ctrl Pts',(3.95096072898711,3.84151718193895,-3.08841088507667));
#9828=CARTESIAN_POINT('Ctrl Pts',(3.03786395995105,3.72693384860553,-4.02073400651229));
#9829=CARTESIAN_POINT('Ctrl Pts',(2.48701127721779,3.66964218193904,-4.39770245315732));
#9830=CARTESIAN_POINT('Ctrl Pts',(1.27766234037718,3.55505884860545,-4.91334639750207));
#9831=CARTESIAN_POINT('Ctrl Pts',(0.619627049962736,3.4977671819386,-5.05178319329073));
#9832=CARTESIAN_POINT('Ctrl Pts',(-0.704706281170879,3.38318384860588,-5.06537827746187));
#9833=CARTESIAN_POINT('Ctrl Pts',(-1.37048327818541,3.32589218193878,-4.94049243718524));
#9834=CARTESIAN_POINT('Ctrl Pts',(-2.60818325905853,3.21130884860571,-4.44253553203559));
#9835=CARTESIAN_POINT('Ctrl Pts',(-3.17960444337468,3.15401718193919,-4.06962455480154));
#9836=CARTESIAN_POINT('Ctrl Pts',(-4.13939783234407,3.03943384860528,-3.1290575182663));
#9837=CARTESIAN_POINT('Ctrl Pts',(-4.52736499532796,2.98214218193882,-2.5617440932366));
#9838=CARTESIAN_POINT('Ctrl Pts',(-5.05787574134119,2.86755884860567,-1.31650352223623));
#9839=CARTESIAN_POINT('Ctrl Pts',(-5.20017477267972,2.81026718193854,-0.639051462402516));
#9840=CARTESIAN_POINT('Ctrl Pts',(-5.21376985687329,2.69568384860595,0.724130693610728));
#9841=CARTESIAN_POINT('Ctrl Pts',(-5.08502178100269,2.638392181939,1.40932446003936));
#9842=CARTESIAN_POINT('Ctrl Pts',(-4.57219807422785,2.52380884860549,2.68291607508254));
#9843=CARTESIAN_POINT('Ctrl Pts',(-4.18828838061282,2.46651718193888,3.27079800167798));
#9844=CARTESIAN_POINT('Ctrl Pts',(-3.22025107658473,2.3519338486056,4.25806165817053));
#9845=CARTESIAN_POINT('Ctrl Pts',(-2.63647690924959,2.29464218193882,4.65702753750094));
#9846=CARTESIAN_POINT('Ctrl Pts',(-1.35534470410106,2.18005884860566,5.20240508517798));
#9847=CARTESIAN_POINT('Ctrl Pts',(-0.658475874835927,2.12276718193851,5.34856635206931));
#9848=CARTESIAN_POINT('Ctrl Pts',(0.743555106044213,2.00818384860598,5.3621614362841));
#9849=CARTESIAN_POINT('Ctrl Pts',(1.44816564189249,1.95089218193886,5.22955112482197));
#9850=CARTESIAN_POINT('Ctrl Pts',(2.75764889110733,1.83630884860562,4.70186061641829));
#9851=CARTESIAN_POINT('Ctrl Pts',(3.36199155998716,1.77901718193906,4.30695220641913));
#9852=CARTESIAN_POINT('Ctrl Pts',(4.37672548399112,1.66443384860542,3.3114446349081));
#9853=CARTESIAN_POINT('Ctrl Pts',(4.78669007967579,1.60714218193865,2.71120972526174));
#9854=CARTESIAN_POINT('Ctrl Pts',(5.3469344290129,1.49255884860583,1.39418588596674));
#9855=CARTESIAN_POINT('Ctrl Pts',(5.49695793145999,1.43526718193912,0.677900287260056));
#9856=CARTESIAN_POINT('Ctrl Pts',(5.51055301569383,1.32068384860537,-0.76297951846838));
#9857=CARTESIAN_POINT('Ctrl Pts',(5.37408046863567,1.26339218193915,-1.4870068237579));
#9858=CARTESIAN_POINT('Ctrl Pts',(4.83152315861431,1.14880884860534,-2.83238170711989));
#9859=CARTESIAN_POINT('Ctrl Pts',(4.42561603222875,1.09151718193863,-3.45318511829405));
#9860=CARTESIAN_POINT('Ctrl Pts',(3.40263819322818,0.976933848605856,-4.49538930981399));
#9861=CARTESIAN_POINT('Ctrl Pts',(2.78594254126256,0.919642181938648,-4.91635262185619));
#9862=CARTESIAN_POINT('Ctrl Pts',(1.43302706784377,0.805058848605838,-5.49146377284226));
#9863=CARTESIAN_POINT('Ctrl Pts',(0.697324699683797,0.747767181938915,-5.64534951085169));
#9864=CARTESIAN_POINT('Ctrl Pts',(-0.782403930892199,0.633183848605571,
-5.65894459510253));
#9865=CARTESIAN_POINT('Ctrl Pts',(-1.5258480056327,0.575892181939075,-5.51860981244762));
#9866=CARTESIAN_POINT('Ctrl Pts',(-2.90711452312302,0.46130884860541,-4.96118570081208));
#9867=CARTESIAN_POINT('Ctrl Pts',(-3.54437866826175,0.404017181938794,-4.5442798657039));
#9868=CARTESIAN_POINT('Ctrl Pts',(-4.07921590611891,0.346725515272242,-4.0190558047933));
#9869=CARTESIAN_POINT('Ctrl Pts',(-2.16033767231584,11.3467255152722,-2.08546000007833));
#9870=CARTESIAN_POINT('Ctrl Pts',(-2.44206781427164,11.2894338486048,-1.81141651031886));
#9871=CARTESIAN_POINT('Ctrl Pts',(-2.67096558433259,11.2321421819387,-1.47966819216879));
#9872=CARTESIAN_POINT('Ctrl Pts',(-2.98550788648136,11.1175588486058,-0.748702056168519));
#9873=CARTESIAN_POINT('Ctrl Pts',(-3.07099283278885,11.0602671819391,-0.349756983242139));
#9874=CARTESIAN_POINT('Ctrl Pts',(-3.0818633980033,10.9456838486053,0.455650002839366));
#9875=CARTESIAN_POINT('Ctrl Pts',(-3.00720596150024,10.8883921819389,0.861795055291616));
#9876=CARTESIAN_POINT('Ctrl Pts',(-2.70531644391264,10.7738088486056,1.61902697886803));
#9877=CARTESIAN_POINT('Ctrl Pts',(-2.47816730458498,10.7165171819386,1.96980110153648));
#9878=CARTESIAN_POINT('Ctrl Pts',(-1.90261007970139,10.6019338486059,2.56073162722495));
#9879=CARTESIAN_POINT('Ctrl Pts',(-1.55440100825198,10.5446421819387,2.80062812645173));
#9880=CARTESIAN_POINT('Ctrl Pts',(-0.787543237963199,10.4300588486058,3.13003723037197));
#9881=CARTESIAN_POINT('Ctrl Pts',(-0.369181395757753,10.3727671819388,3.21938441215601));
#9882=CARTESIAN_POINT('Ctrl Pts',(0.475074415355009,10.2581838486057,3.23025497743655));
#9883=CARTESIAN_POINT('Ctrl Pts',(0.900636237067393,10.2008921819389,3.15173530532716));
#9884=CARTESIAN_POINT('Ctrl Pts',(1.69375979497017,10.0863088486056,2.83497898609545));
#9885=CARTESIAN_POINT('Ctrl Pts',(2.0609946597737,10.029017181939,2.59683113043342));
#9886=CARTESIAN_POINT('Ctrl Pts',(2.67939545311748,9.91443384860552,1.99380363798266));
#9887=CARTESIAN_POINT('Ctrl Pts',(2.93029066857928,9.8571421819389,1.62913382432459));
#9888=CARTESIAN_POINT('Ctrl Pts',(3.27456657425417,9.74255884860558,0.826384419768452));
#9889=CARTESIAN_POINT('Ctrl Pts',(3.36777599152708,9.68526718193864,0.388605808260406));
#9890=CARTESIAN_POINT('Ctrl Pts',(3.37864655686589,9.57068384860584,-0.49449882785769));
#9891=CARTESIAN_POINT('Ctrl Pts',(3.29626464915295,9.51339218193913,-0.939477418855915));
#9892=CARTESIAN_POINT('Ctrl Pts',(2.96464152827939,9.39880884860535,-1.76849261105957));
#9893=CARTESIAN_POINT('Ctrl Pts',(2.71549495627589,9.34151718193865,-2.15218821802195));
#9894=CARTESIAN_POINT('Ctrl Pts',(2.0849971962699,9.22693384860583,-2.79805927899898));
#9895=CARTESIAN_POINT('Ctrl Pts',(1.70386664038741,9.1696421819387,-3.05995321071421));
#9896=CARTESIAN_POINT('Ctrl Pts',(0.865225601583496,9.05505884860578,-3.419095918129));
#9897=CARTESIAN_POINT('Ctrl Pts',(0.408030220752219,8.99776718193874,-3.51616757090102));
#9898=CARTESIAN_POINT('Ctrl Pts',(-0.513923240349536,8.88318384860575,-3.52703813629236));
#9899=CARTESIAN_POINT('Ctrl Pts',(-0.978318600655415,8.82589218193907,-3.44079399297743));
#9900=CARTESIAN_POINT('Ctrl Pts',(-1.84322542713799,8.71130884860541,-3.09430407046464));
#9901=CARTESIAN_POINT('Ctrl Pts',(-2.24338177627905,8.65401718193906,-2.8341587821133));
#9902=CARTESIAN_POINT('Ctrl Pts',(-2.91672310487163,8.53943384860543,-2.1761907545622));
#9903=CARTESIAN_POINT('Ctrl Pts',(-3.18961575285625,8.48214218193879,-1.77859945644224));
#9904=CARTESIAN_POINT('Ctrl Pts',(-3.56362526199671,8.36755884860569,-0.904066783406526));
#9905=CARTESIAN_POINT('Ctrl Pts',(-3.66455915027763,8.3102671819386,-0.427454633233268));
#9906=CARTESIAN_POINT('Ctrl Pts',(-3.67542971571615,8.19568384860588,0.533347652830617));
#9907=CARTESIAN_POINT('Ctrl Pts',(-3.58532333680026,8.13839218193865,1.01715978246527));
#9908=CARTESIAN_POINT('Ctrl Pts',(-3.22396661265153,8.02380884860583,1.91795824320607));
#9909=CARTESIAN_POINT('Ctrl Pts',(-2.95282260794454,7.96651718193906,2.33457533454633));
#9910=CARTESIAN_POINT('Ctrl Pts',(-2.26738431286067,7.85193384860543,3.03538693073411));
#9911=CARTESIAN_POINT('Ctrl Pts',(-1.85333227248862,7.79464218193892,3.31927829500387));
#9912=CARTESIAN_POINT('Ctrl Pts',(-0.942907965238003,7.68005884860556,3.70815460585884));
#9913=CARTESIAN_POINT('Ctrl Pts',(-0.446879045704217,7.62276718193853,3.81295072965703));
#9914=CARTESIAN_POINT('Ctrl Pts',(0.552772065301601,7.50818384860596,3.82382129513715));
#9915=CARTESIAN_POINT('Ctrl Pts',(1.05600096428514,7.45089218193902,3.7298526806217));
#9916=CARTESIAN_POINT('Ctrl Pts',(1.99269105926411,7.33630884860546,3.35362915483982));
#9917=CARTESIAN_POINT('Ctrl Pts',(2.42576889282071,7.27901718193947,3.07148643377194));
#9918=CARTESIAN_POINT('Ctrl Pts',(3.15405075658949,7.16443384860501,2.35857787116297));
#9919=CARTESIAN_POINT('Ctrl Pts',(3.4489408371573,7.10714218193936,1.92806508852736));
#9920=CARTESIAN_POINT('Ctrl Pts',(3.85268394971518,6.99255884860513,0.981749147077123));
#9921=CARTESIAN_POINT('Ctrl Pts',(3.96134230903857,6.93526718193912,0.466303458167944));
#9922=CARTESIAN_POINT('Ctrl Pts',(3.97221287455602,6.82068384860537,-0.572196477765365));
#9923=CARTESIAN_POINT('Ctrl Pts',(3.87438202444231,6.76339218193869,-1.09484214611198));
#9924=CARTESIAN_POINT('Ctrl Pts',(3.48329169702894,6.6488088486058,-2.06742387531521));
#9925=CARTESIAN_POINT('Ctrl Pts',(3.19015025959274,6.5915171819388,-2.51696245110363));
#9926=CARTESIAN_POINT('Ctrl Pts',(2.44977142947187,6.47693384860569,-3.27271458243633));
#9927=CARTESIAN_POINT('Ctrl Pts',(2.00279790455941,6.41964218193941,-3.57860337931556));
#9928=CARTESIAN_POINT('Ctrl Pts',(1.02059032892293,6.30505884860508,-3.99721329356667));
#9929=CARTESIAN_POINT('Ctrl Pts',(0.485727870620802,6.24776718193879,-4.10973388842147));
#9930=CARTESIAN_POINT('Ctrl Pts',(-0.591620890218261,6.1331838486057,-4.12060445397352));
#9931=CARTESIAN_POINT('Ctrl Pts',(-1.13368332795069,6.07589218193929,-4.01891136825983));
#9932=CARTESIAN_POINT('Ctrl Pts',(-2.14215669135443,5.9613088486052,-3.61295423922114));
#9933=CARTESIAN_POINT('Ctrl Pts',(-2.60815600939102,5.90401718193932,-3.30881408541235));
#9934=CARTESIAN_POINT('Ctrl Pts',(-3.39137840827869,5.78943384860516,-2.54096498778195));
#9935=CARTESIAN_POINT('Ctrl Pts',(-3.70826592147772,5.73214218193892,-2.07753072058528));
#9936=CARTESIAN_POINT('Ctrl Pts',(-4.14174263741426,5.61755884860556,-1.05943151077492));
#9937=CARTESIAN_POINT('Ctrl Pts',(-4.25812546780629,5.56026718193889,-0.505152283069884));
#9938=CARTESIAN_POINT('Ctrl Pts',(-4.26899603338911,5.44568384860559,0.611045302667398));
#9939=CARTESIAN_POINT('Ctrl Pts',(-4.16344071207717,5.38839218193887,1.17252450979444));
#9940=CARTESIAN_POINT('Ctrl Pts',(-3.74261678141353,5.27380884860562,2.21688950738861));
#9941=CARTESIAN_POINT('Ctrl Pts',(-3.4274779112251,5.21651718193883,2.69934956768717));
#9942=CARTESIAN_POINT('Ctrl Pts',(-2.63215854609891,5.10193384860566,3.5100422341123));
#9943=CARTESIAN_POINT('Ctrl Pts',(-2.15226353660435,5.04464218193881,3.83792846364419));
#9944=CARTESIAN_POINT('Ctrl Pts',(-1.0982726926337,4.93005884860567,4.28627198125755));
#9945=CARTESIAN_POINT('Ctrl Pts',(-0.524576695510519,4.87276718193882,4.40651704719262));
#9946=CARTESIAN_POINT('Ctrl Pts',(0.630469715108076,4.75818384860566,4.41738761280318));
#9947=CARTESIAN_POINT('Ctrl Pts',(1.21136569164331,4.70089218193903,4.30797005589403));
#9948=CARTESIAN_POINT('Ctrl Pts',(2.29162232341768,4.58630884860546,3.87227932360639));
#9949=CARTESIAN_POINT('Ctrl Pts',(2.79054312598678,4.529017181939,3.5461417370364));
#9950=CARTESIAN_POINT('Ctrl Pts',(3.62870605994246,4.41443384860549,2.72335210441731));
#9951=CARTESIAN_POINT('Ctrl Pts',(3.96759100581396,4.35714218193895,2.22699635262072));
#9952=CARTESIAN_POINT('Ctrl Pts',(4.43080132509753,4.24255884860554,1.13711387449518));
#9953=CARTESIAN_POINT('Ctrl Pts',(4.55490862657983,4.18526718193866,0.544001107941954));
#9954=CARTESIAN_POINT('Ctrl Pts',(4.56577919221637,4.07068384860583,-0.649894127539557));
#9955=CARTESIAN_POINT('Ctrl Pts',(4.45249939970698,4.01339218193886,-1.25020687350361));
#9956=CARTESIAN_POINT('Ctrl Pts',(4.00194186580315,3.89880884860562,-2.36635513943533));
#9957=CARTESIAN_POINT('Ctrl Pts',(3.66480556284339,3.84151718193895,-2.88173668429245));
#9958=CARTESIAN_POINT('Ctrl Pts',(2.81454566274002,3.72693384860553,-3.74736988576655));
#9959=CARTESIAN_POINT('Ctrl Pts',(2.30172916862896,3.66964218193904,-4.09725354798759));
#9960=CARTESIAN_POINT('Ctrl Pts',(1.17595505636478,3.55505884860545,-4.57533066893367));
#9961=CARTESIAN_POINT('Ctrl Pts',(0.563425520373289,3.4977671819386,-4.70330020596852));
#9962=CARTESIAN_POINT('Ctrl Pts',(-0.669318539970923,3.38318384860588,-4.71417077162809));
#9963=CARTESIAN_POINT('Ctrl Pts',(-1.28904805536363,3.32589218193878,-4.59702874352091));
#9964=CARTESIAN_POINT('Ctrl Pts',(-2.44108795545323,3.21130884860571,-4.13160440799895));
#9965=CARTESIAN_POINT('Ctrl Pts',(-2.97293024260301,3.15401718193919,-3.78346938864651));
#9966=CARTESIAN_POINT('Ctrl Pts',(-3.86603371158577,3.03943384860528,-2.90573922106659));
#9967=CARTESIAN_POINT('Ctrl Pts',(-4.22691609016478,2.98214218193882,-2.37646198463267));
#9968=CARTESIAN_POINT('Ctrl Pts',(-4.71986001276623,2.86755884860567,-1.21479623823893));
#9969=CARTESIAN_POINT('Ctrl Pts',(-4.8516917853577,2.81026718193854,-0.582849932796644));
#9970=CARTESIAN_POINT('Ctrl Pts',(-4.86256235103931,2.69568384860595,0.688742952394343));
#9971=CARTESIAN_POINT('Ctrl Pts',(-4.74155808733321,2.638392181939,1.32788923723221));
#9972=CARTESIAN_POINT('Ctrl Pts',(-4.26126695019637,2.52380884860549,2.5158207714626));
#9973=CARTESIAN_POINT('Ctrl Pts',(-3.90213321444713,2.46651718193888,3.06412380091759));
#9974=CARTESIAN_POINT('Ctrl Pts',(-2.99693277939567,2.3519338486056,3.98469753740094));
#9975=CARTESIAN_POINT('Ctrl Pts',(-2.45119480063163,2.29464218193882,4.35657863234452));
#9976=CARTESIAN_POINT('Ctrl Pts',(-1.2536374201178,2.18005884860566,4.86438935659626));
#9977=CARTESIAN_POINT('Ctrl Pts',(-0.602274345215141,2.12276718193851,5.00008336474837));
#9978=CARTESIAN_POINT('Ctrl Pts',(0.708167364812911,2.00818384860598,5.01095393044905));
#9979=CARTESIAN_POINT('Ctrl Pts',(1.36673041909958,1.95089218193886,4.8860874311467));
#9980=CARTESIAN_POINT('Ctrl Pts',(2.59055358747315,1.83630884860562,4.39092949239261));
#9981=CARTESIAN_POINT('Ctrl Pts',(3.15531735923718,1.77901718193906,4.02079704024371));
#9982=CARTESIAN_POINT('Ctrl Pts',(4.10336136321113,1.66443384860542,3.08812633772876));
#9983=CARTESIAN_POINT('Ctrl Pts',(4.48624117452488,1.60714218193865,2.52592761663043));
#9984=CARTESIAN_POINT('Ctrl Pts',(5.00891870042567,1.49255884860583,1.29247860199682));
#9985=CARTESIAN_POINT('Ctrl Pts',(5.14847494413939,1.43526718193912,0.621698757625503));
#9986=CARTESIAN_POINT('Ctrl Pts',(5.15934550985844,1.32068384860537,-0.727591777223308));
#9987=CARTESIAN_POINT('Ctrl Pts',(5.0306167749558,1.26339218193915,-1.40557160097741));
#9988=CARTESIAN_POINT('Ctrl Pts',(4.52059203459322,1.14880884860534,-2.66528640347329));
#9989=CARTESIAN_POINT('Ctrl Pts',(4.13946086604337,1.09151718193863,-3.24651091755445));
#9990=CARTESIAN_POINT('Ctrl Pts',(3.17931989605881,0.976933848605856,-4.22202518902362));
#9991=CARTESIAN_POINT('Ctrl Pts',(2.60066043261983,0.919642181938648,-4.61590371671046));
#9992=CARTESIAN_POINT('Ctrl Pts',(1.33131978388528,0.805058848605838,-5.15344804424985));
#9993=CARTESIAN_POINT('Ctrl Pts',(0.641123170036348,0.747767181938915,-5.29686652353057));
#9994=CARTESIAN_POINT('Ctrl Pts',(-0.747016189634228,0.633183848605571,
-5.30773708926766));
#9995=CARTESIAN_POINT('Ctrl Pts',(-1.44441278286383,0.575892181939075,-5.17514611876316));
#9996=CARTESIAN_POINT('Ctrl Pts',(-2.74001921946479,0.46130884860541,-4.65025457679559));
#9997=CARTESIAN_POINT('Ctrl Pts',(-3.33770446803392,0.404017181938794,-4.25812469903555));
#9998=CARTESIAN_POINT('Ctrl Pts',(-3.83919674535392,0.346725515272242,-3.76431907311593));
#9999=CARTESIAN_POINT('Ctrl Pts',(-2.12557398216503,11.,-2.11821519670878));
#10000=CARTESIAN_POINT('Ctrl Pts',(-2.41159176945725,10.9427083333325,-1.84872226348015));
#10001=CARTESIAN_POINT('Ctrl Pts',(-2.6456803034859,10.8854166666664,-1.52067018109149));
#10002=CARTESIAN_POINT('Ctrl Pts',(-2.97162798586693,10.7708333333336,-0.794830755283512));
#10003=CARTESIAN_POINT('Ctrl Pts',(-3.06332306119362,10.7135416666669,-0.397314139662748));
#10004=CARTESIAN_POINT('Ctrl Pts',(-3.08669273082211,10.5989583333331,0.407721033857582));
#10005=CARTESIAN_POINT('Ctrl Pts',(-3.01831935235521,10.5416666666666,0.814922877330024));
#10006=CARTESIAN_POINT('Ctrl Pts',(-2.728119788021,10.4270833333334,1.57659449107116));
#10007=CARTESIAN_POINT('Ctrl Pts',(-2.50637194487625,10.3697916666664,1.93074976622997));
#10008=CARTESIAN_POINT('Ctrl Pts',(-1.93991583267103,10.2552083333337,2.53025558222984));
#10009=CARTESIAN_POINT('Ctrl Pts',(-1.59540299717169,10.1979166666664,2.77534284559852));
#10010=CARTESIAN_POINT('Ctrl Pts',(-0.833671937081177,10.0833333333336,
3.11615732976406));
#10011=CARTESIAN_POINT('Ctrl Pts',(-0.416738552178117,10.0260416666666,
3.21171464055396));
#10012=CARTESIAN_POINT('Ctrl Pts',(0.427145446372979,9.91145833333345,3.23508431026218));
#10013=CARTESIAN_POINT('Ctrl Pts',(0.853764059103477,9.85416666666669,3.16284869617602));
#10014=CARTESIAN_POINT('Ctrl Pts',(1.65132730717562,9.73958333333332,2.85778233020993));
#10015=CARTESIAN_POINT('Ctrl Pts',(2.02194332446279,9.68229166666673,2.62503577071995));
#10016=CARTESIAN_POINT('Ctrl Pts',(2.64891940812677,9.56770833333328,2.03110939095704));
#10017=CARTESIAN_POINT('Ctrl Pts',(2.9050053877204,9.51041666666666,1.67013581324179));
#10018=CARTESIAN_POINT('Ctrl Pts',(3.26068667365192,9.39583333333334,0.872513118888943));
#10019=CARTESIAN_POINT('Ctrl Pts',(3.36010621991895,9.3385416666664,0.436162964680591));
#10020=CARTESIAN_POINT('Ctrl Pts',(3.38347588969759,9.22395833333361,-0.446569858875482));
#10021=CARTESIAN_POINT('Ctrl Pts',(3.30737803999626,9.16666666666689,-0.892605240889856));
#10022=CARTESIAN_POINT('Ctrl Pts',(2.98744487239941,9.05208333333312,-1.72606012326716));
#10023=CARTESIAN_POINT('Ctrl Pts',(2.74369959655829,8.99479166666641,-2.11313688270712));
#10024=CARTESIAN_POINT('Ctrl Pts',(2.1223029492484,8.8802083333336,-2.76758323401219));
#10025=CARTESIAN_POINT('Ctrl Pts',(1.74486862930228,8.82291666666647,-3.03466792985017));
#10026=CARTESIAN_POINT('Ctrl Pts',(0.911354300706321,8.70833333333354,-3.40521601753191));
#10027=CARTESIAN_POINT('Ctrl Pts',(0.455587377172263,8.6510416666665,-3.5084977992874));
#10028=CARTESIAN_POINT('Ctrl Pts',(-0.465994271367186,8.53645833333351,
-3.53186746912954));
#10029=CARTESIAN_POINT('Ctrl Pts',(-0.93144642268745,8.47916666666683,-3.45190738381581));
#10030=CARTESIAN_POINT('Ctrl Pts',(-1.80079293934749,8.36458333333318,-3.11710741458959));
#10031=CARTESIAN_POINT('Ctrl Pts',(-2.20433044096071,8.30729166666683,-2.86236342239196));
#10032=CARTESIAN_POINT('Ctrl Pts',(-2.88624705988836,8.1927083333332,-2.21349650754444));
#10033=CARTESIAN_POINT('Ctrl Pts',(-3.1643304719878,8.13541666666656,-1.81960144535507));
#10034=CARTESIAN_POINT('Ctrl Pts',(-3.54974536140404,8.02083333333345,-0.950195482531384));
#10035=CARTESIAN_POINT('Ctrl Pts',(-3.65688937865929,7.96354166666637,-0.475011789653154));
#10036=CARTESIAN_POINT('Ctrl Pts',(-3.68025904855805,7.84895833333365,0.485418683848109));
#10037=CARTESIAN_POINT('Ctrl Pts',(-3.59643672763413,7.79166666666665,0.970287604495667));
#10038=CARTESIAN_POINT('Ctrl Pts',(-3.246769956781,7.67708333333337,1.8755257554172));
#10039=CARTESIAN_POINT('Ctrl Pts',(-2.98102724821984,7.61979166666659,2.29552399922486));
#10040=CARTESIAN_POINT('Ctrl Pts',(-2.30469006584627,7.50520833333343,3.00491088575395));
#10041=CARTESIAN_POINT('Ctrl Pts',(-1.89433426139971,7.44791666666668,3.29399301413121));
#10042=CARTESIAN_POINT('Ctrl Pts',(-0.989036664364609,7.33333333333333,
3.69427470527038));
#10043=CARTESIAN_POINT('Ctrl Pts',(-0.49443620212397,7.27604166666629,3.80528095803426));
#10044=CARTESIAN_POINT('Ctrl Pts',(0.50484309631896,7.16145833333372,3.82865062798349));
#10045=CARTESIAN_POINT('Ctrl Pts',(1.00912878631411,7.10416666666678,3.74096607145172));
#10046=CARTESIAN_POINT('Ctrl Pts',(1.95025857147667,6.98958333333323,3.37643249897315));
#10047=CARTESIAN_POINT('Ctrl Pts',(2.38671755749636,6.93229166666724,3.09969107404422));
#10048=CARTESIAN_POINT('Ctrl Pts',(3.12357471161222,6.81770833333277,2.39588362415159));
#10049=CARTESIAN_POINT('Ctrl Pts',(3.42365555628099,6.76041666666712,1.96906707743673));
#10050=CARTESIAN_POINT('Ctrl Pts',(3.83880404913035,6.64583333333289,1.02787784620545));
#10051=CARTESIAN_POINT('Ctrl Pts',(3.95367253741186,6.58854166666688,0.51386061458762));
#10052=CARTESIAN_POINT('Ctrl Pts',(3.97704220740629,6.47395833333313,-0.524267508782646));
#10053=CARTESIAN_POINT('Ctrl Pts',(3.88549541526866,6.41666666666645,-1.04796996813959));
#10054=CARTESIAN_POINT('Ctrl Pts',(3.50609504116593,6.30208333333356,-2.02499138752914));
#10055=CARTESIAN_POINT('Ctrl Pts',(3.2183548998624,6.24479166666656,-2.47791111577681));
#10056=CARTESIAN_POINT('Ctrl Pts',(2.48707718246311,6.13020833333345,-3.24223853746153));
#10057=CARTESIAN_POINT('Ctrl Pts',(2.04379989346725,6.07291666666717,-3.55331809843599));
#10058=CARTESIAN_POINT('Ctrl Pts',(1.06671902805278,5.95833333333284,-3.9833333929851));
#10059=CARTESIAN_POINT('Ctrl Pts',(0.533285027040294,5.90104166666655,-4.10206411679133));
#10060=CARTESIAN_POINT('Ctrl Pts',(-0.543691921235359,5.78645833333346,
-4.12543378682723));
#10061=CARTESIAN_POINT('Ctrl Pts',(-1.08681114997705,5.72916666666705,-4.03002475908303));
#10062=CARTESIAN_POINT('Ctrl Pts',(-2.0997242035696,5.61458333333296,-3.63575758336128));
#10063=CARTESIAN_POINT('Ctrl Pts',(-2.56910467406188,5.55729166666709,-3.33701872567955));
#10064=CARTESIAN_POINT('Ctrl Pts',(-3.36090236330622,5.44270833333292,-2.57827074077566));
#10065=CARTESIAN_POINT('Ctrl Pts',(-3.68298064059524,5.38541666666669,-2.11853270949184));
#10066=CARTESIAN_POINT('Ctrl Pts',(-4.12786273683561,5.27083333333332,-1.10556020990605));
#10067=CARTESIAN_POINT('Ctrl Pts',(-4.25045569617289,5.21354166666665,-0.552709439489368));
#10068=CARTESIAN_POINT('Ctrl Pts',(-4.27382536624608,5.09895833333335,0.563116333684488));
#10069=CARTESIAN_POINT('Ctrl Pts',(-4.17455410289751,5.04166666666663,1.12565233181968));
#10070=CARTESIAN_POINT('Ctrl Pts',(-3.76542012555652,4.92708333333338,2.17445701960491));
#10071=CARTESIAN_POINT('Ctrl Pts',(-3.45568255149002,4.86979166666659,2.66029823235588));
#10072=CARTESIAN_POINT('Ctrl Pts',(-2.6694642990949,4.75520833333342,3.47956618914197));
#10073=CARTESIAN_POINT('Ctrl Pts',(-2.19326552550957,4.69791666666658,3.81264318275876));
#10074=CARTESIAN_POINT('Ctrl Pts',(-1.14440139176617,4.58333333333343,4.27239208068185));
#10075=CARTESIAN_POINT('Ctrl Pts',(-0.572133851929879,4.52604166666658,
4.39884727555618));
#10076=CARTESIAN_POINT('Ctrl Pts',(0.582540746125043,4.41145833333343,4.42221694566319));
#10077=CARTESIAN_POINT('Ctrl Pts',(1.16449351366757,4.35416666666679,4.31908344671154));
#10078=CARTESIAN_POINT('Ctrl Pts',(2.24918983563495,4.23958333333322,3.89508266775222));
#10079=CARTESIAN_POINT('Ctrl Pts',(2.75149179065353,4.18229166666676,3.57434637729919));
#10080=CARTESIAN_POINT('Ctrl Pts',(3.59823001497408,4.06770833333325,2.76065785741543));
#10081=CARTESIAN_POINT('Ctrl Pts',(3.94230572492611,4.01041666666671,2.26799834152485));
#10082=CARTESIAN_POINT('Ctrl Pts',(4.41692142452426,3.8958333333333,1.18324257362874));
#10083=CARTESIAN_POINT('Ctrl Pts',(4.54723885494094,3.83854166666642,0.591558264361257));
#10084=CARTESIAN_POINT('Ctrl Pts',(4.57060852507883,3.72395833333359,-0.601965158556466));
#10085=CARTESIAN_POINT('Ctrl Pts',(4.46361279052205,3.66666666666662,-1.20333469552689));
#10086=CARTESIAN_POINT('Ctrl Pts',(4.02474520995143,3.55208333333339,-2.32392265165357));
#10087=CARTESIAN_POINT('Ctrl Pts',(3.69301020310442,3.49479166666671,-2.84268534895739));
#10088=CARTESIAN_POINT('Ctrl Pts',(2.85185141573989,3.38020833333329,-3.71689384079999));
#10089=CARTESIAN_POINT('Ctrl Pts',(2.34273115753217,3.3229166666668,-4.07196826709743));
#10090=CARTESIAN_POINT('Ctrl Pts',(1.22208375549926,3.20833333333321,-4.56145076836271));
#10091=CARTESIAN_POINT('Ctrl Pts',(0.610982676792531,3.15104166666636,-4.6956304343271));
#10092=CARTESIAN_POINT('Ctrl Pts',(-0.621389570987771,3.03645833333365,
-4.71900010449308));
#10093=CARTESIAN_POINT('Ctrl Pts',(-1.24217587738614,2.97916666666654,-4.60814213433379));
#10094=CARTESIAN_POINT('Ctrl Pts',(-2.39865546767225,2.86458333333347,-4.15440775214941));
#10095=CARTESIAN_POINT('Ctrl Pts',(-2.93387890726637,2.80729166666695,-3.81167402890586));
#10096=CARTESIAN_POINT('Ctrl Pts',(-3.83555766662078,2.69270833333305,-2.94304497406814));
#10097=CARTESIAN_POINT('Ctrl Pts',(-4.20163080927273,2.63541666666658,-2.41746397353493));
#10098=CARTESIAN_POINT('Ctrl Pts',(-4.70598011219716,2.52083333333343,-1.26092493737436));
#10099=CARTESIAN_POINT('Ctrl Pts',(-4.84402201371418,2.4635416666663,-0.630407089215845));
#10100=CARTESIAN_POINT('Ctrl Pts',(-4.86739168390641,2.34895833333371,0.64081398341115));
#10101=CARTESIAN_POINT('Ctrl Pts',(-4.75267147814405,2.29166666666676,1.28101705925391));
#10102=CARTESIAN_POINT('Ctrl Pts',(-4.28407029434887,2.17708333333325,2.47338828368244));
#10103=CARTESIAN_POINT('Ctrl Pts',(-3.93033785470491,2.11979166666664,3.0250724655795));
#10104=CARTESIAN_POINT('Ctrl Pts',(-3.0342385323988,2.00520833333337,3.95422149243741));
#10105=CARTESIAN_POINT('Ctrl Pts',(-2.49219678953305,1.94791666666658,4.33129335145034));
#10106=CARTESIAN_POINT('Ctrl Pts',(-1.29976611925407,1.83333333333343,4.85050945602931));
#10107=CARTESIAN_POINT('Ctrl Pts',(-0.6498315016342,1.77604166666627,4.99241359310244));
#10108=CARTESIAN_POINT('Ctrl Pts',(0.660238395829575,1.66145833333374,5.01578326331855));
#10109=CARTESIAN_POINT('Ctrl Pts',(1.31985824112059,1.60416666666663,4.89720082195578));
#10110=CARTESIAN_POINT('Ctrl Pts',(2.54812109969368,1.48958333333338,4.41373283654687));
#10111=CARTESIAN_POINT('Ctrl Pts',(3.1162660238978,1.43229166666683,4.04900168050008));
#10112=CARTESIAN_POINT('Ctrl Pts',(4.07288531824889,1.31770833333318,3.1254320907333));
#10113=CARTESIAN_POINT('Ctrl Pts',(4.460955893629,1.26041666666641,2.56692960553103));
#10114=CARTESIAN_POINT('Ctrl Pts',(4.99503879986042,1.1458333333336,1.33860730113391));
#10115=CARTESIAN_POINT('Ctrl Pts',(5.14080517249185,1.08854166666688,0.669255914044516));
#10116=CARTESIAN_POINT('Ctrl Pts',(5.16417484272955,0.973958333333134,-0.679662808239928));
#10117=CARTESIAN_POINT('Ctrl Pts',(5.04173016576313,0.916666666666909,-1.35869942299763));
#10118=CARTESIAN_POINT('Ctrl Pts',(4.54339537874923,0.8020833333331,-2.62285391569459));
#10119=CARTESIAN_POINT('Ctrl Pts',(4.16766550629842,0.744791666666392,-3.20745958221381));
#10120=CARTESIAN_POINT('Ctrl Pts',(3.21662564906467,0.630208333333619,-4.19154914406263));
#10121=CARTESIAN_POINT('Ctrl Pts',(2.6416624215197,0.572916666666411,-4.59061843581319));
#10122=CARTESIAN_POINT('Ctrl Pts',(1.3774484830231,0.4583333333336,-5.13956814368599));
#10123=CARTESIAN_POINT('Ctrl Pts',(0.688680326455284,0.401041666666677,
-5.28919675188146));
#10124=CARTESIAN_POINT('Ctrl Pts',(-0.69908722065077,0.286458333333334,
-5.31256642214034));
#10125=CARTESIAN_POINT('Ctrl Pts',(-1.39754060488348,0.229166666666838,
-5.1862595095691));
#10126=CARTESIAN_POINT('Ctrl Pts',(-2.69758673168668,0.114583333333173,
-4.67305792095299));
#10127=CARTESIAN_POINT('Ctrl Pts',(-3.29865313262765,0.0572916666665569,
-4.28632933922004));
#10128=CARTESIAN_POINT('Ctrl Pts',(-3.80443305520312,5.20417042793042E-15,
-3.79707426974638));
#10129=CARTESIAN_POINT('Ctrl Pts',(-2.09081029201422,10.6532744847278,-2.15097039333923));
#10130=CARTESIAN_POINT('Ctrl Pts',(-2.38111572464286,10.5959828180603,-1.88602801664143));
#10131=CARTESIAN_POINT('Ctrl Pts',(-2.6203950226392,10.5386911513942,-1.56167217001419));
#10132=CARTESIAN_POINT('Ctrl Pts',(-2.9577480852525,10.4241078180613,-0.840959454398505));
#10133=CARTESIAN_POINT('Ctrl Pts',(-3.05565328959838,10.3668161513947,-0.444871296083357));
#10134=CARTESIAN_POINT('Ctrl Pts',(-3.09152206364091,10.2522328180609,0.359792064875797));
#10135=CARTESIAN_POINT('Ctrl Pts',(-3.02943274321019,10.1949411513944,0.768050699368431));
#10136=CARTESIAN_POINT('Ctrl Pts',(-2.75092313212936,10.0803578180611,1.53416200327429));
#10137=CARTESIAN_POINT('Ctrl Pts',(-2.53457658516751,10.0230661513941,1.89169843092347));
#10138=CARTESIAN_POINT('Ctrl Pts',(-1.97722158564067,9.90848281806141,2.49977953723472));
#10139=CARTESIAN_POINT('Ctrl Pts',(-1.6364049860914,9.8511911513942,2.75005756474531));
#10140=CARTESIAN_POINT('Ctrl Pts',(-0.879800636199156,9.73660781806133,
3.10227742915614));
#10141=CARTESIAN_POINT('Ctrl Pts',(-0.46429570859848,9.67931615139432,3.2040448689519));
#10142=CARTESIAN_POINT('Ctrl Pts',(0.379216477390949,9.56473281806121,3.2399136430878));
#10143=CARTESIAN_POINT('Ctrl Pts',(0.806891881139562,9.50744115139445,3.17396208702488));
#10144=CARTESIAN_POINT('Ctrl Pts',(1.60889481938107,9.39285781806108,2.8805856743244));
#10145=CARTESIAN_POINT('Ctrl Pts',(1.98289198915187,9.33556615139449,2.65324041100648));
#10146=CARTESIAN_POINT('Ctrl Pts',(2.61844336313606,9.22098281806105,2.06841514393141));
#10147=CARTESIAN_POINT('Ctrl Pts',(2.87972010686153,9.16369115139443,1.71113780215899));
#10148=CARTESIAN_POINT('Ctrl Pts',(3.24680677304967,9.0491078180611,0.918641818009435));
#10149=CARTESIAN_POINT('Ctrl Pts',(3.35243644831083,8.99181615139416,0.483720121100777));
#10150=CARTESIAN_POINT('Ctrl Pts',(3.38830522252928,8.87723281806137,-0.398640889893273));
#10151=CARTESIAN_POINT('Ctrl Pts',(3.31849143083958,8.81994115139465,-0.845733062923796));
#10152=CARTESIAN_POINT('Ctrl Pts',(3.01024821651943,8.70535781806088,-1.68362763547476));
#10153=CARTESIAN_POINT('Ctrl Pts',(2.77190423684068,8.64806615139417,-2.0740855473923));
#10154=CARTESIAN_POINT('Ctrl Pts',(2.15960870222691,8.53348281806136,-2.73710718902539));
#10155=CARTESIAN_POINT('Ctrl Pts',(1.78587061821714,8.47619115139423,-3.00938264898613));
#10156=CARTESIAN_POINT('Ctrl Pts',(0.957482999829145,8.36160781806131,-3.39133611693482));
#10157=CARTESIAN_POINT('Ctrl Pts',(0.503144533592307,8.30431615139426,-3.50082802767378));
#10158=CARTESIAN_POINT('Ctrl Pts',(-0.418065302384836,8.18973281806127,
-3.53669680196673));
#10159=CARTESIAN_POINT('Ctrl Pts',(-0.884574244719486,8.13244115139459,
-3.4630207746542));
#10160=CARTESIAN_POINT('Ctrl Pts',(-1.75836045155699,8.01785781806094,-3.13991075871454));
#10161=CARTESIAN_POINT('Ctrl Pts',(-2.16527910564236,7.96056615139459,-2.89056806267063));
#10162=CARTESIAN_POINT('Ctrl Pts',(-2.85577101490508,7.84598281806096,-2.25080226052667));
#10163=CARTESIAN_POINT('Ctrl Pts',(-3.13904519111934,7.78869115139432,-1.8606034342679));
#10164=CARTESIAN_POINT('Ctrl Pts',(-3.53586546081137,7.67410781806122,-0.996324181656243));
#10165=CARTESIAN_POINT('Ctrl Pts',(-3.64921960704095,7.61681615139413,-0.52256894607304));
#10166=CARTESIAN_POINT('Ctrl Pts',(-3.68508838139996,7.50223281806141,0.437489714865601));
#10167=CARTESIAN_POINT('Ctrl Pts',(-3.60755011846799,7.44494115139464,0.923415426526065));
#10168=CARTESIAN_POINT('Ctrl Pts',(-3.26957330091048,7.33035781806089,1.83309326762834));
#10169=CARTESIAN_POINT('Ctrl Pts',(-3.00923188849514,7.27306615139411,2.25647266390339));
#10170=CARTESIAN_POINT('Ctrl Pts',(-2.34199581883187,7.15848281806142,2.9744348407738));
#10171=CARTESIAN_POINT('Ctrl Pts',(-1.93533625031079,7.10119115139444,3.26870773325855));
#10172=CARTESIAN_POINT('Ctrl Pts',(-1.03516536349121,6.98660781806109,3.68039480468192));
#10173=CARTESIAN_POINT('Ctrl Pts',(-0.541993358543724,6.92931615139405,
3.79761118641148));
#10174=CARTESIAN_POINT('Ctrl Pts',(0.45691412733632,6.81473281806148,3.83347996082984));
#10175=CARTESIAN_POINT('Ctrl Pts',(0.962256608343087,6.75744115139454,3.75207946228173));
#10176=CARTESIAN_POINT('Ctrl Pts',(1.90782608368924,6.64285781806099,3.39923584310647));
#10177=CARTESIAN_POINT('Ctrl Pts',(2.34766622217201,6.585566151395,3.12789571431651));
#10178=CARTESIAN_POINT('Ctrl Pts',(3.09309866663495,6.47098281806054,2.4331893771402));
#10179=CARTESIAN_POINT('Ctrl Pts',(3.39837027540469,6.41369115139488,2.01006906634609));
#10180=CARTESIAN_POINT('Ctrl Pts',(3.82492414854553,6.29910781806065,1.07400654533378));
#10181=CARTESIAN_POINT('Ctrl Pts',(3.94600276578516,6.24181615139464,0.561417771007294));
#10182=CARTESIAN_POINT('Ctrl Pts',(3.98187154025657,6.1272328180609,-0.476338539799928));
#10183=CARTESIAN_POINT('Ctrl Pts',(3.89660880609501,6.06994115139421,-1.00109779016719));
#10184=CARTESIAN_POINT('Ctrl Pts',(3.52889838530292,5.95535781806132,-1.98255889974307));
#10185=CARTESIAN_POINT('Ctrl Pts',(3.24655954013207,5.89806615139432,-2.43885978044999));
#10186=CARTESIAN_POINT('Ctrl Pts',(2.52438293545435,5.78348281806122,-3.21176249248673));
#10187=CARTESIAN_POINT('Ctrl Pts',(2.08480188237509,5.72619115139493,-3.52803281755643));
#10188=CARTESIAN_POINT('Ctrl Pts',(1.11284772718263,5.6116078180606,-3.96945349240354));
#10189=CARTESIAN_POINT('Ctrl Pts',(0.580842183459787,5.55431615139431,-4.0943943451612));
#10190=CARTESIAN_POINT('Ctrl Pts',(-0.495762952252458,5.43973281806122,
-4.13026311968094));
#10191=CARTESIAN_POINT('Ctrl Pts',(-1.03993897200342,5.38244115139481,-4.04113814990623));
#10192=CARTESIAN_POINT('Ctrl Pts',(-2.05729171578477,5.26785781806072,-3.65856092750142));
#10193=CARTESIAN_POINT('Ctrl Pts',(-2.53005333873273,5.21056615139485,-3.36522336594676));
#10194=CARTESIAN_POINT('Ctrl Pts',(-3.33042631833374,5.09598281806069,-2.61557649376936));
#10195=CARTESIAN_POINT('Ctrl Pts',(-3.65769535971276,5.03869115139445,-2.1595346983984));
#10196=CARTESIAN_POINT('Ctrl Pts',(-4.11398283625697,4.92410781806109,-1.15168890903718));
#10197=CARTESIAN_POINT('Ctrl Pts',(-4.24278592453948,4.86681615139442,-0.600266595908851));
#10198=CARTESIAN_POINT('Ctrl Pts',(-4.27865469910306,4.75223281806112,0.515187364701578));
#10199=CARTESIAN_POINT('Ctrl Pts',(-4.18566749371785,4.69494115139439,1.07878015384492));
#10200=CARTESIAN_POINT('Ctrl Pts',(-3.78822346969952,4.58035781806114,2.13202453182121));
#10201=CARTESIAN_POINT('Ctrl Pts',(-3.48388719175493,4.52306615139435,2.62124689702459));
#10202=CARTESIAN_POINT('Ctrl Pts',(-2.70677005209088,4.40848281806118,3.44909014417165));
#10203=CARTESIAN_POINT('Ctrl Pts',(-2.2342675144148,4.35119115139434,3.78735790187333));
#10204=CARTESIAN_POINT('Ctrl Pts',(-1.19053009089864,4.2366078180612,4.25851218010615));
#10205=CARTESIAN_POINT('Ctrl Pts',(-0.61969100834924,4.17931615139434,4.39117750391975));
#10206=CARTESIAN_POINT('Ctrl Pts',(0.53461177714201,4.06473281806119,4.42704627852319));
#10207=CARTESIAN_POINT('Ctrl Pts',(1.11762133569182,4.00744115139456,4.33019683752905));
#10208=CARTESIAN_POINT('Ctrl Pts',(2.20675734785223,3.89285781806098,3.91788601189805));
#10209=CARTESIAN_POINT('Ctrl Pts',(2.71244045532029,3.83556615139452,3.60255101756198));
#10210=CARTESIAN_POINT('Ctrl Pts',(3.56775397000571,3.72098281806102,2.79796361041354));
#10211=CARTESIAN_POINT('Ctrl Pts',(3.91702044403826,3.66369115139447,2.30900033042897));
#10212=CARTESIAN_POINT('Ctrl Pts',(4.40304152395098,3.54910781806106,1.22937127276231));
#10213=CARTESIAN_POINT('Ctrl Pts',(4.53956908330205,3.49181615139418,0.63911542078056));
#10214=CARTESIAN_POINT('Ctrl Pts',(4.5754378579413,3.37723281806136,-0.554036189573376));
#10215=CARTESIAN_POINT('Ctrl Pts',(4.47472618133712,3.31994115139439,-1.15646251755018));
#10216=CARTESIAN_POINT('Ctrl Pts',(4.0475485540997,3.20535781806115,-2.28149016387182));
#10217=CARTESIAN_POINT('Ctrl Pts',(3.72121484336545,3.14806615139448,-2.80363401362233));
#10218=CARTESIAN_POINT('Ctrl Pts',(2.88915716873977,3.03348281806106,-3.68641779583343));
#10219=CARTESIAN_POINT('Ctrl Pts',(2.38373314643537,2.97619115139456,-4.04668298620726));
#10220=CARTESIAN_POINT('Ctrl Pts',(1.26821245463375,2.86160781806097,-4.54757086779175));
#10221=CARTESIAN_POINT('Ctrl Pts',(0.658539833211772,2.80431615139412,-4.68796066268569));
#10222=CARTESIAN_POINT('Ctrl Pts',(-0.573460602004618,2.68973281806141,
-4.72382943735807));
#10223=CARTESIAN_POINT('Ctrl Pts',(-1.19530369940865,2.6324411513943,-4.61925552514667));
#10224=CARTESIAN_POINT('Ctrl Pts',(-2.35622297989128,2.51785781806124,-4.17721109629987));
#10225=CARTESIAN_POINT('Ctrl Pts',(-2.89482757192974,2.46056615139471,-3.83987866916521));
#10226=CARTESIAN_POINT('Ctrl Pts',(-3.8050816216558,2.34598281806081,-2.98035072706969));
#10227=CARTESIAN_POINT('Ctrl Pts',(-4.17634552838067,2.28869115139434,-2.4584659624372));
#10228=CARTESIAN_POINT('Ctrl Pts',(-4.6921002116281,2.1741078180612,-1.30705363650978));
#10229=CARTESIAN_POINT('Ctrl Pts',(-4.83635224207065,2.11681615139406,-0.677964245635046));
#10230=CARTESIAN_POINT('Ctrl Pts',(-4.87222101677351,2.00223281806147,0.592885014427957));
#10231=CARTESIAN_POINT('Ctrl Pts',(-4.76378486895489,1.94494115139452,1.23414488127561));
#10232=CARTESIAN_POINT('Ctrl Pts',(-4.30687363850137,1.83035781806102,2.43095579590227));
#10233=CARTESIAN_POINT('Ctrl Pts',(-3.95854249496268,1.77306615139441,2.98602113024142));
#10234=CARTESIAN_POINT('Ctrl Pts',(-3.07154428540192,1.65848281806113,3.92374544747388));
#10235=CARTESIAN_POINT('Ctrl Pts',(-2.53319877843447,1.60119115139435,4.30600807055617));
#10236=CARTESIAN_POINT('Ctrl Pts',(-1.34589481839034,1.48660781806119,4.83662955546236));
#10237=CARTESIAN_POINT('Ctrl Pts',(-0.697388658053259,1.42931615139403,
4.9847438214565));
#10238=CARTESIAN_POINT('Ctrl Pts',(0.61230942684624,1.3147328180615,5.02061259618806));
#10239=CARTESIAN_POINT('Ctrl Pts',(1.27298606314159,1.25744115139439,4.90831421276487));
#10240=CARTESIAN_POINT('Ctrl Pts',(2.50568861191421,1.14285781806115,4.43653618070112));
#10241=CARTESIAN_POINT('Ctrl Pts',(3.07721468855841,1.08556615139459,4.07720632075644));
#10242=CARTESIAN_POINT('Ctrl Pts',(4.04240927328666,0.970982818060947,3.16273784373784));
#10243=CARTESIAN_POINT('Ctrl Pts',(4.43567061273313,0.913691151394175,2.60793159443164));
#10244=CARTESIAN_POINT('Ctrl Pts',(4.98115889929517,0.79910781806136,1.384736000271));
#10245=CARTESIAN_POINT('Ctrl Pts',(5.13313540084431,0.741816151394642,0.716813070463529));
#10246=CARTESIAN_POINT('Ctrl Pts',(5.16900417560066,0.627232818060896,-0.631733839256547));
#10247=CARTESIAN_POINT('Ctrl Pts',(5.05284355657047,0.569941151394671,-1.31182724501786));
#10248=CARTESIAN_POINT('Ctrl Pts',(4.56619872290524,0.455357818060863,-2.5804214279159));
#10249=CARTESIAN_POINT('Ctrl Pts',(4.19587014655347,0.398066151394155,-3.16840824687318));
#10250=CARTESIAN_POINT('Ctrl Pts',(3.25393140207052,0.283482818061382,-4.16107309910165));
#10251=CARTESIAN_POINT('Ctrl Pts',(2.68266441041957,0.226191151394174,-4.56533315491593));
#10252=CARTESIAN_POINT('Ctrl Pts',(1.42357718216092,0.111607818061363,-5.12568824312213));
#10253=CARTESIAN_POINT('Ctrl Pts',(0.736237482874218,0.0543161513944401,
-5.28152698023234));
#10254=CARTESIAN_POINT('Ctrl Pts',(-0.651158251667311,-0.0602671819389035,
-5.31739575501303));
#10255=CARTESIAN_POINT('Ctrl Pts',(-1.35066842690312,-0.117558848605399,
-5.19737290037505));
#10256=CARTESIAN_POINT('Ctrl Pts',(-2.65515424390857,-0.232142181939065,
-4.69586126511038));
#10257=CARTESIAN_POINT('Ctrl Pts',(-3.25960179722137,-0.28943384860568,
-4.31453397940454));
#10258=CARTESIAN_POINT('Ctrl Pts',(-3.76966936505231,-0.346725515272232,
-3.82982946637684));
#10259=CARTESIAN_POINT('Ctrl Pts',(-2.33082945277919,10.6532744847278,-2.40570712501662));
#10260=CARTESIAN_POINT('Ctrl Pts',(-2.65447984657204,10.5959828180603,-2.10934631273779));
#10261=CARTESIAN_POINT('Ctrl Pts',(-2.92084392795166,10.5386911513942,-1.74695427828554));
#10262=CARTESIAN_POINT('Ctrl Pts',(-3.29576381367816,10.4241078180613,-0.942666738728405));
#10263=CARTESIAN_POINT('Ctrl Pts',(-3.40413627693083,10.3668161513947,-0.501072825334149));
#10264=CARTESIAN_POINT('Ctrl Pts',(-3.44272956946446,10.2522328180609,0.39517980573707));
#10265=CARTESIAN_POINT('Ctrl Pts',(-3.37289643675743,10.1949411513944,0.849485922498689));
#10266=CARTESIAN_POINT('Ctrl Pts',(-3.06185425628309,10.0803578180611,1.70125730657109));
#10267=CARTESIAN_POINT('Ctrl Pts',(-2.82073175110235,10.0230661513941,2.0983726319291));
#10268=CARTESIAN_POINT('Ctrl Pts',(-2.2005398830606,9.90848281806141,2.77314365775904));
#10269=CARTESIAN_POINT('Ctrl Pts',(-1.82168709441022,9.8511911513942,3.05050647003645));
#10270=CARTESIAN_POINT('Ctrl Pts',(-0.98150792048159,9.73660781806133,3.44029315760313));
#10271=CARTESIAN_POINT('Ctrl Pts',(-0.520497237899657,9.67931615139432,
3.55252785628273));
#10272=CARTESIAN_POINT('Ctrl Pts',(0.41460421830261,9.56473281806121,3.59112114891296));
#10273=CARTESIAN_POINT('Ctrl Pts',(0.888327104224163,9.50744115139445,3.51742578058933));
#10274=CARTESIAN_POINT('Ctrl Pts',(1.77599012272354,9.39285781806108,3.19151679846092));
#10275=CARTESIAN_POINT('Ctrl Pts',(2.18956619012306,9.33556615139449,2.93939557697384));
#10276=CARTESIAN_POINT('Ctrl Pts',(2.89180748369484,9.22098281806105,2.29173344131881));
#10277=CARTESIAN_POINT('Ctrl Pts',(3.18016901213384,9.16369115139443,1.8964199105197));
#10278=CARTESIAN_POINT('Ctrl Pts',(3.58482250151549,9.0491078180611,1.02034910224998));
#10279=CARTESIAN_POINT('Ctrl Pts',(3.70091943564033,8.99181615139416,0.539921650446381));
#10280=CARTESIAN_POINT('Ctrl Pts',(3.73951272835577,8.87723281806137,-0.434028630849363));
#10281=CARTESIAN_POINT('Ctrl Pts',(3.66195512441954,8.81994115139465,-0.927168285967855));
#10282=CARTESIAN_POINT('Ctrl Pts',(3.32117934064045,8.70535781806088,-1.85072293885776));
#10283=CARTESIAN_POINT('Ctrl Pts',(3.05805940283662,8.64806615139417,-2.28075974833291));
#10284=CARTESIAN_POINT('Ctrl Pts',(2.38292699958574,8.53348281806136,-3.01047130961474));
#10285=CARTESIAN_POINT('Ctrl Pts',(1.97115272661516,8.47619115139423,-3.30983155424184));
#10286=CARTESIAN_POINT('Ctrl Pts',(1.05919028403238,8.36160781806131,-3.72935184541724));
#10287=CARTESIAN_POINT('Ctrl Pts',(0.559346062977528,8.30431615139426,-3.8493110150021));
#10288=CARTESIAN_POINT('Ctrl Pts',(-0.453453043380547,8.18973281806127,
-3.8879043077944));
#10289=CARTESIAN_POINT('Ctrl Pts',(-0.966009467727636,8.13244115139459,
-3.80648446824784));
#10290=CARTESIAN_POINT('Ctrl Pts',(-1.92545575497591,8.01785781806094,-3.45084188282187));
#10291=CARTESIAN_POINT('Ctrl Pts',(-2.37195330655562,7.96056615139459,-3.17672322869252));
#10292=CARTESIAN_POINT('Ctrl Pts',(-3.12913513552178,7.84598281806096,-2.47412055785955));
#10293=CARTESIAN_POINT('Ctrl Pts',(-3.43949409635991,7.78869115139432,-2.04588554269906));
#10294=CARTESIAN_POINT('Ctrl Pts',(-3.87388118930893,7.67410781806122,-1.09803146582633));
#10295=CARTESIAN_POINT('Ctrl Pts',(-3.9977025943682,7.61681615139413,-0.578770475493801));
#10296=CARTESIAN_POINT('Ctrl Pts',(-4.03629588722871,7.50223281806141,0.472877455896854));
#10297=CARTESIAN_POINT('Ctrl Pts',(-3.95101381207413,7.44494115139464,1.00485064950196));
#10298=CARTESIAN_POINT('Ctrl Pts',(-3.58050442500531,7.33035781806089,2.00018857107951));
#10299=CARTESIAN_POINT('Ctrl Pts',(-3.29538705454006,7.27306615139411,2.46314686479214));
#10300=CARTESIAN_POINT('Ctrl Pts',(-2.56531411614172,7.15848281806142,3.24779896141502));
#10301=CARTESIAN_POINT('Ctrl Pts',(-2.12061835877177,7.10119115139444,3.5691566384858));
#10302=CARTESIAN_POINT('Ctrl Pts',(-1.13687264763148,6.98660781806109,4.01841053319279));
#10303=CARTESIAN_POINT('Ctrl Pts',(-0.598194887996293,6.92931615139405,
4.14609417373796));
#10304=CARTESIAN_POINT('Ctrl Pts',(0.492301868399383,6.81473281806148,4.18468746665935));
#10305=CARTESIAN_POINT('Ctrl Pts',(1.04369183128993,6.75744115139454,4.09554315589853));
#10306=CARTESIAN_POINT('Ctrl Pts',(2.07492138716947,6.64285781806099,3.71016696719063));
#10307=CARTESIAN_POINT('Ctrl Pts',(2.55434042303921,6.585566151395,3.41405088038211));
#10308=CARTESIAN_POINT('Ctrl Pts',(3.36646278729771,6.47098281806054,2.65650767442937));
#10309=CARTESIAN_POINT('Ctrl Pts',(3.69881918061998,6.41369115139488,2.19535117483371));
#10310=CARTESIAN_POINT('Ctrl Pts',(4.16293987706837,6.29910781806065,1.1757138294474));
#10311=CARTESIAN_POINT('Ctrl Pts',(4.29448575311062,6.24181615139464,0.617619300488533));
#10312=CARTESIAN_POINT('Ctrl Pts',(4.3330790460871,6.1272328180609,-0.511726280891663));
#10313=CARTESIAN_POINT('Ctrl Pts',(4.24007249972198,6.06994115139421,-1.0825330130876));
#10314=CARTESIAN_POINT('Ctrl Pts',(3.8398295093769,5.95535781806132,-2.14965420324974));
#10315=CARTESIAN_POINT('Ctrl Pts',(3.53271470621635,5.89806615139432,-2.64553398129709));
#10316=CARTESIAN_POINT('Ctrl Pts',(2.74770123272482,5.78348281806122,-3.48512661316959));
#10317=CARTESIAN_POINT('Ctrl Pts',(2.27008399088731,5.72619115139493,-3.82848172276042));
#10318=CARTESIAN_POINT('Ctrl Pts',(1.21455501127165,5.6116078180606,-4.30746922093769));
#10319=CARTESIAN_POINT('Ctrl Pts',(0.637043712966868,5.55431615139431,-4.44287733248579));
#10320=CARTESIAN_POINT('Ctrl Pts',(-0.531150693370039,5.43973281806122,
-4.48147062551234));
#10321=CARTESIAN_POINT('Ctrl Pts',(-1.12137419490063,5.38244115139481,-4.38460184354212));
#10322=CARTESIAN_POINT('Ctrl Pts',(-2.22438701931463,5.26785781806072,-3.96949205156649));
#10323=CARTESIAN_POINT('Ctrl Pts',(-2.73672753956158,5.21056615139485,-3.651378532048));
#10324=CARTESIAN_POINT('Ctrl Pts',(-3.60379043903486,5.09598281806069,-2.83889479102288));
#10325=CARTESIAN_POINT('Ctrl Pts',(-3.95814426490714,5.03869115139445,-2.34481680693236));
#10326=CARTESIAN_POINT('Ctrl Pts',(-4.45199856480073,4.92410781806109,-1.25339619310446));
#10327=CARTESIAN_POINT('Ctrl Pts',(-4.59126891186371,4.86681615139442,-0.656468125439367));
#10328=CARTESIAN_POINT('Ctrl Pts',(-4.62986220493482,4.75223281806112,0.550575105842595));
#10329=CARTESIAN_POINT('Ctrl Pts',(-4.52913118736181,4.69494115139439,1.1602153767205));
#10330=CARTESIAN_POINT('Ctrl Pts',(-4.09915459375653,4.58035781806114,2.2991198353727));
#10331=CARTESIAN_POINT('Ctrl Pts',(-3.77004235787144,4.52306615139435,2.82792109783747));
#10332=CARTESIAN_POINT('Ctrl Pts',(-2.93008834932913,4.40848281806118,3.72245426488873));
#10333=CARTESIAN_POINT('Ctrl Pts',(-2.41954962296883,4.35119115139434,4.08780680705904));
#10334=CARTESIAN_POINT('Ctrl Pts',(-1.29223737494584,4.2366078180612,4.59652790865858));
#10335=CARTESIAN_POINT('Ctrl Pts',(-0.675892537901207,4.17931615139434,
4.73966049124288));
#10336=CARTESIAN_POINT('Ctrl Pts',(0.569999518304482,4.06473281806119,4.77825378435605));
#10337=CARTESIAN_POINT('Ctrl Pts',(1.19905655854802,4.00744115139456,4.67366053118015));
#10338=CARTESIAN_POINT('Ctrl Pts',(2.37385265142312,3.89285781806098,4.2288171359479));
#10339=CARTESIAN_POINT('Ctrl Pts',(2.91911465611821,3.83556615139452,3.88870618369294));
#10340=CARTESIAN_POINT('Ctrl Pts',(3.84111809073775,3.72098281806102,3.02128190763733));
#10341=CARTESIAN_POINT('Ctrl Pts',(4.21746934921548,3.66369115139447,2.49428243900129));
#10342=CARTESIAN_POINT('Ctrl Pts',(4.74105725251191,3.54910781806106,1.33107855679123));
#10343=CARTESIAN_POINT('Ctrl Pts',(4.88805207062498,3.49181615139418,0.695316950351842));
#10344=CARTESIAN_POINT('Ctrl Pts',(4.92664536377436,3.37723281806136,-0.589423930755165));
#10345=CARTESIAN_POINT('Ctrl Pts',(4.81818987499502,3.31994115139439,-1.23789774038871));
#10346=CARTESIAN_POINT('Ctrl Pts',(4.35847967814275,3.20535781806115,-2.44858546746038));
#10347=CARTESIAN_POINT('Ctrl Pts',(4.00737000950903,3.14806615139448,-3.01030821440669));
#10348=CARTESIAN_POINT('Ctrl Pts',(3.11247546595094,3.03348281806106,-3.95978191657904));
#10349=CARTESIAN_POINT('Ctrl Pts',(2.56901525502413,2.97619115139456,-4.34713189137729));
#10350=CARTESIAN_POINT('Ctrl Pts',(1.36991973864622,2.86160781806097,-4.88558659635986));
#10351=CARTESIAN_POINT('Ctrl Pts',(0.714741362801074,2.80431615139412,-5.0364436500079));
#10352=CARTESIAN_POINT('Ctrl Pts',(-0.608848343204429,2.68973281806141,
-5.07503694319185));
#10353=CARTESIAN_POINT('Ctrl Pts',(-1.27673892223029,2.6324411513943,-4.96271921881158));
#10354=CARTESIAN_POINT('Ctrl Pts',(-2.52331828349673,2.51785781806124,-4.48814222033592));
#10355=CARTESIAN_POINT('Ctrl Pts',(-3.10150177270171,2.46056615139471,-4.12603383532024));
#10356=CARTESIAN_POINT('Ctrl Pts',(-4.0784457424138,2.34598281806081,-3.20366902426941));
#10357=CARTESIAN_POINT('Ctrl Pts',(-4.47679443354355,2.28869115139434,-2.64374807104099));
#10358=CARTESIAN_POINT('Ctrl Pts',(-5.03011594020335,2.1741078180612,-1.40876092050723));
#10359=CARTESIAN_POINT('Ctrl Pts',(-5.18483522939207,2.11681615139406,-0.734165775240769));
#10360=CARTESIAN_POINT('Ctrl Pts',(-5.22342852260808,2.00223281806147,0.628272755644193));
#10361=CARTESIAN_POINT('Ctrl Pts',(-5.10724856262497,1.94494115139452,1.31558010408276));
#10362=CARTESIAN_POINT('Ctrl Pts',(-4.61780476253225,1.83035781806102,2.59805109952221));
#10363=CARTESIAN_POINT('Ctrl Pts',(-4.24469766112837,1.77306615139441,3.1926953310021));
#10364=CARTESIAN_POINT('Ctrl Pts',(-3.29486258259099,1.65848281806113,4.19710956824316));
#10365=CARTESIAN_POINT('Ctrl Pts',(-2.71848088705236,1.60119115139435,4.60645697571289));
#10366=CARTESIAN_POINT('Ctrl Pts',(-1.44760210237368,1.48660781806119,5.17464528404378));
#10367=CARTESIAN_POINT('Ctrl Pts',(-0.753590187674045,1.42931615139403,
5.33322680877775));
#10368=CARTESIAN_POINT('Ctrl Pts',(0.647697168077543,1.3147328180615,5.37182010202281));
#10369=CARTESIAN_POINT('Ctrl Pts',(1.35442128593412,1.25744115139439,5.25177790643984));
#10370=CARTESIAN_POINT('Ctrl Pts',(2.67278391554878,1.14285781806115,4.7474673047271));
#10371=CARTESIAN_POINT('Ctrl Pts',(3.28388888930855,1.08556615139459,4.36336148693201));
#10372=CARTESIAN_POINT('Ctrl Pts',(4.3157733940665,0.970982818060947,3.38605614091702));
#10373=CARTESIAN_POINT('Ctrl Pts',(4.73611951788435,0.913691151394175,2.79321370306255));
#10374=CARTESIAN_POINT('Ctrl Pts',(5.31917462788209,0.79910781806136,1.48644328424131));
#10375=CARTESIAN_POINT('Ctrl Pts',(5.48161838816491,0.741816151394642,0.773014600098004));
#10376=CARTESIAN_POINT('Ctrl Pts',(5.52021168143606,0.627232818060896,-0.667121580501539));
#10377=CARTESIAN_POINT('Ctrl Pts',(5.39630725025002,0.569941151394671,-1.39326246779836));
#10378=CARTESIAN_POINT('Ctrl Pts',(4.87712984692664,0.455357818060863,-2.7475167315625));
#10379=CARTESIAN_POINT('Ctrl Pts',(4.48202531273885,0.398066151394155,-3.37508244761294));
#10380=CARTESIAN_POINT('Ctrl Pts',(3.47724969923989,0.283482818061382,-4.43443721989186));
#10381=CARTESIAN_POINT('Ctrl Pts',(2.8679465190623,0.226191151394174,-4.86578206006134));
#10382=CARTESIAN_POINT('Ctrl Pts',(1.52528446611942,0.111607818061363,-5.46370397171486));
#10383=CARTESIAN_POINT('Ctrl Pts',(0.792439012521748,0.0543161513944402,
-5.63000996755282));
#10384=CARTESIAN_POINT('Ctrl Pts',(-0.686545992925361,-0.0602671819389035,
-5.66860326084855));
#10385=CARTESIAN_POINT('Ctrl Pts',(-1.43210364967231,-0.117558848605399,
-5.54083659405887));
#10386=CARTESIAN_POINT('Ctrl Pts',(-2.82224954756648,-0.232142181939065,
-5.00679238912752));
#10387=CARTESIAN_POINT('Ctrl Pts',(-3.46627599744854,-0.28943384860568,
-4.6006891460729));
#10388=CARTESIAN_POINT('Ctrl Pts',(-4.0096885258173,-0.346725515272232,
-4.08456619805421));
#10389=CARTESIAN_POINT('Ctrl Pts',(-2.36559314293001,11.,-2.37295192838617));
#10390=CARTESIAN_POINT('Ctrl Pts',(-2.68495589138643,10.9427083333325,-2.0720405595763));
#10391=CARTESIAN_POINT('Ctrl Pts',(-2.94612920879841,10.8854166666664,-1.70595228936294));
#10392=CARTESIAN_POINT('Ctrl Pts',(-3.30964371429254,10.7708333333336,-0.896538039613314));
#10393=CARTESIAN_POINT('Ctrl Pts',(-3.41180604852602,10.7135416666669,-0.453515668913589));
#10394=CARTESIAN_POINT('Ctrl Pts',(-3.4379002366457,10.5989583333331,0.443108774718904));
#10395=CARTESIAN_POINT('Ctrl Pts',(-3.36178304590245,10.5416666666666,0.896358100460257));
#10396=CARTESIAN_POINT('Ctrl Pts',(-3.03905091217473,10.4270833333334,1.74368979436799));
#10397=CARTESIAN_POINT('Ctrl Pts',(-2.79252711081109,10.3697916666664,2.13742396723561));
#10398=CARTESIAN_POINT('Ctrl Pts',(-2.16323413009096,10.2552083333337,2.80361970275416));
#10399=CARTESIAN_POINT('Ctrl Pts',(-1.78068510549046,10.1979166666664,3.07579175088966));
#10400=CARTESIAN_POINT('Ctrl Pts',(-0.935379221363662,10.0833333333336,
3.45417305821104));
#10401=CARTESIAN_POINT('Ctrl Pts',(-0.472940081479242,10.0260416666666,
3.56019762788479));
#10402=CARTESIAN_POINT('Ctrl Pts',(0.462533187284589,9.91145833333345,3.58629181608734));
#10403=CARTESIAN_POINT('Ctrl Pts',(0.935199282188079,9.85416666666669,3.50631238974053));
#10404=CARTESIAN_POINT('Ctrl Pts',(1.81842261051809,9.73958333333332,3.16871345434639));
#10405=CARTESIAN_POINT('Ctrl Pts',(2.22861752543397,9.68229166666673,2.91119093668731));
#10406=CARTESIAN_POINT('Ctrl Pts',(2.92228352868554,9.56770833333328,2.25442768834444));
#10407=CARTESIAN_POINT('Ctrl Pts',(3.20545429299277,9.51041666666666,1.85541792160244));
#10408=CARTESIAN_POINT('Ctrl Pts',(3.59870240211769,9.39583333333334,0.974220403129539));
#10409=CARTESIAN_POINT('Ctrl Pts',(3.70858920724845,9.3385416666664,0.492364494026195));
#10410=CARTESIAN_POINT('Ctrl Pts',(3.73468339552408,9.22395833333361,-0.481957599831572));
#10411=CARTESIAN_POINT('Ctrl Pts',(3.65084173357628,9.16666666666689,-0.974040463933888));
#10412=CARTESIAN_POINT('Ctrl Pts',(3.29837599652037,9.05208333333312,-1.8931554266502));
#10413=CARTESIAN_POINT('Ctrl Pts',(3.02985476255422,8.99479166666641,-2.31981108364774));
#10414=CARTESIAN_POINT('Ctrl Pts',(2.34562124660724,8.8802083333336,-3.04094735460153));
#10415=CARTESIAN_POINT('Ctrl Pts',(1.93015073770027,8.82291666666647,-3.33511683510577));
#10416=CARTESIAN_POINT('Ctrl Pts',(1.01306158490958,8.70833333333354,-3.74323174601444));
#10417=CARTESIAN_POINT('Ctrl Pts',(0.511788906557484,8.6510416666665,-3.85698078661577));
#10418=CARTESIAN_POINT('Ctrl Pts',(-0.501382012362897,8.53645833333351,
-3.88307497495716));
#10419=CARTESIAN_POINT('Ctrl Pts',(-1.01288164569554,8.47916666666683,-3.79537107740945));
#10420=CARTESIAN_POINT('Ctrl Pts',(-1.96788824276646,8.36458333333318,-3.42803853869692));
#10421=CARTESIAN_POINT('Ctrl Pts',(-2.41100464187403,8.30729166666683,-3.14851858841386));
#10422=CARTESIAN_POINT('Ctrl Pts',(-3.159611180505,8.1927083333332,-2.43681480487731));
#10423=CARTESIAN_POINT('Ctrl Pts',(-3.46477937722837,8.13541666666656,-2.00488355378617));
#10424=CARTESIAN_POINT('Ctrl Pts',(-3.8877610899016,8.02083333333345,-1.05190276670153));
#10425=CARTESIAN_POINT('Ctrl Pts',(-4.00537236598643,7.96354166666637,-0.531213319073915));
#10426=CARTESIAN_POINT('Ctrl Pts',(-4.03146655438691,7.84895833333365,0.520806424879362));
#10427=CARTESIAN_POINT('Ctrl Pts',(-3.93990042124014,7.79166666666665,1.05172282747159));
#10428=CARTESIAN_POINT('Ctrl Pts',(-3.55770108087595,7.67708333333337,2.04262105886835));
#10429=CARTESIAN_POINT('Ctrl Pts',(-3.26718241426475,7.61979166666659,2.50219820011361));
#10430=CARTESIAN_POINT('Ctrl Pts',(-2.52800836315612,7.50520833333343,3.27827500639517));
#10431=CARTESIAN_POINT('Ctrl Pts',(-2.07961636986072,7.44791666666668,3.59444191935829));
#10432=CARTESIAN_POINT('Ctrl Pts',(-1.09074394850484,7.33333333333333,4.03229043378143));
#10433=CARTESIAN_POINT('Ctrl Pts',(-0.550637731576509,7.27604166666629,
4.15376394536062));
#10434=CARTESIAN_POINT('Ctrl Pts',(0.540230837381994,7.16145833333372,4.17985813381312));
#10435=CARTESIAN_POINT('Ctrl Pts',(1.09056400926098,7.10416666666678,4.08442976506864));
#10436=CARTESIAN_POINT('Ctrl Pts',(2.11735387495688,6.98958333333323,3.68736362305719));
#10437=CARTESIAN_POINT('Ctrl Pts',(2.59339175836345,6.93229166666724,3.38584624010982));
#10438=CARTESIAN_POINT('Ctrl Pts',(3.3969388322751,6.81770833333277,2.61920192144075));
#10439=CARTESIAN_POINT('Ctrl Pts',(3.72410446149635,6.76041666666712,2.15434918592434));
#10440=CARTESIAN_POINT('Ctrl Pts',(4.17681977765313,6.64583333333289,1.12958513031907));
#10441=CARTESIAN_POINT('Ctrl Pts',(4.30215552473732,6.58854166666688,0.570062144068889));
#10442=CARTESIAN_POINT('Ctrl Pts',(4.32824971323683,6.47395833333313,-0.559655249874413));
#10443=CARTESIAN_POINT('Ctrl Pts',(4.22895910889563,6.41666666666645,-1.12940519106012));
#10444=CARTESIAN_POINT('Ctrl Pts',(3.81702616523991,6.30208333333356,-2.19208669103568));
#10445=CARTESIAN_POINT('Ctrl Pts',(3.50451006594675,6.24479166666656,-2.68458531662391));
#10446=CARTESIAN_POINT('Ctrl Pts',(2.71039547973352,6.13020833333345,-3.51560265814439));
#10447=CARTESIAN_POINT('Ctrl Pts',(2.22908200197935,6.07291666666717,-3.85376700363998));
#10448=CARTESIAN_POINT('Ctrl Pts',(1.16842631214193,5.95833333333284,-4.32134912151925));
#10449=CARTESIAN_POINT('Ctrl Pts',(0.589486556547344,5.90104166666655,-4.45054710411593));
#10450=CARTESIAN_POINT('Ctrl Pts',(-0.579079662352908,5.78645833333346,
-4.47664129265863));
#10451=CARTESIAN_POINT('Ctrl Pts',(-1.16824637287424,5.72916666666705,-4.37348845271886));
#10452=CARTESIAN_POINT('Ctrl Pts',(-2.26681950709949,5.61458333333296,-3.94668870742641));
#10453=CARTESIAN_POINT('Ctrl Pts',(-2.77577887489086,5.55729166666709,-3.62317389178086));
#10454=CARTESIAN_POINT('Ctrl Pts',(-3.6342664840072,5.44270833333292,-2.80158903802911));
#10455=CARTESIAN_POINT('Ctrl Pts',(-3.98342954578962,5.38541666666669,-2.30381481802579));
#10456=CARTESIAN_POINT('Ctrl Pts',(-4.46587846537937,5.27083333333332,-1.20726749397333));
#10457=CARTESIAN_POINT('Ctrl Pts',(-4.59893868349712,5.21354166666665,-0.608910969019916));
#10458=CARTESIAN_POINT('Ctrl Pts',(-4.62503287207784,5.09895833333335,0.598504074825539));
#10459=CARTESIAN_POINT('Ctrl Pts',(-4.51801779654147,5.04166666666663,1.20708755469526));
#10460=CARTESIAN_POINT('Ctrl Pts',(-4.07635124961353,4.92708333333338,2.34155232315641));
#10461=CARTESIAN_POINT('Ctrl Pts',(-3.74183771760646,4.86979166666659,2.86697243316876));
#10462=CARTESIAN_POINT('Ctrl Pts',(-2.89278259633321,4.75520833333342,3.75293030985906));
#10463=CARTESIAN_POINT('Ctrl Pts',(-2.37854763406351,4.69791666666658,4.1130920879442));
#10464=CARTESIAN_POINT('Ctrl Pts',(-1.24610867581347,4.58333333333343,4.61040780923455));
#10465=CARTESIAN_POINT('Ctrl Pts',(-0.628335381481812,4.52604166666658,
4.74733026287932));
#10466=CARTESIAN_POINT('Ctrl Pts',(0.617928487287482,4.41145833333343,4.77342445149605));
#10467=CARTESIAN_POINT('Ctrl Pts',(1.24592873652376,4.35416666666679,4.66254714036264));
#10468=CARTESIAN_POINT('Ctrl Pts',(2.41628513920584,4.23958333333322,4.20601379180208));
#10469=CARTESIAN_POINT('Ctrl Pts',(2.95816599145146,4.18229166666676,3.86050154342994));
#10470=CARTESIAN_POINT('Ctrl Pts',(3.87159413570613,4.06770833333325,2.98397615463943));
#10471=CARTESIAN_POINT('Ctrl Pts',(4.24275463010319,4.01041666666671,2.45328045009706));
#10472=CARTESIAN_POINT('Ctrl Pts',(4.75493715308532,3.8958333333333,1.28494985765777));
#10473=CARTESIAN_POINT('Ctrl Pts',(4.89572184226387,3.83854166666642,0.647759793932574));
#10474=CARTESIAN_POINT('Ctrl Pts',(4.9218160309119,3.72395833333359,-0.637352899738291));
#10475=CARTESIAN_POINT('Ctrl Pts',(4.80707648417982,3.66666666666662,-1.28476991836542));
#10476=CARTESIAN_POINT('Ctrl Pts',(4.33567633399462,3.55208333333339,-2.49101795524214));
#10477=CARTESIAN_POINT('Ctrl Pts',(3.97916536924807,3.49479166666671,-3.04935954974168));
#10478=CARTESIAN_POINT('Ctrl Pts',(3.075169712951,3.38020833333329,-3.99025796154567));
#10479=CARTESIAN_POINT('Ctrl Pts',(2.52801326612096,3.3229166666668,-4.37241717226731));
#10480=CARTESIAN_POINT('Ctrl Pts',(1.3237910395117,3.20833333333321,-4.89946649693097));
#10481=CARTESIAN_POINT('Ctrl Pts',(0.667184206381905,3.15104166666636,-5.04411342164931));
#10482=CARTESIAN_POINT('Ctrl Pts',(-0.656777312187654,3.03645833333365,
-5.07020761032686));
#10483=CARTESIAN_POINT('Ctrl Pts',(-1.32361110020785,2.97916666666654,-4.95160582799841));
#10484=CARTESIAN_POINT('Ctrl Pts',(-2.56575077127763,2.86458333333347,-4.46533887618575));
#10485=CARTESIAN_POINT('Ctrl Pts',(-3.1405531080382,2.80729166666695,-4.09782919506089));
#10486=CARTESIAN_POINT('Ctrl Pts',(-4.10892178737893,2.69270833333305,-3.16636327126786));
#10487=CARTESIAN_POINT('Ctrl Pts',(-4.50207971443576,2.63541666666658,-2.60274608213879));
#10488=CARTESIAN_POINT('Ctrl Pts',(-5.04399584077227,2.52083333333343,-1.36263222137173));
#10489=CARTESIAN_POINT('Ctrl Pts',(-5.1925050010359,2.4635416666663,-0.686608618821642));
#10490=CARTESIAN_POINT('Ctrl Pts',(-5.21859918974068,2.34895833333371,0.67620172462746));
#10491=CARTESIAN_POINT('Ctrl Pts',(-5.09613517181383,2.29166666666676,1.36245228206106));
#10492=CARTESIAN_POINT('Ctrl Pts',(-4.59500141838005,2.17708333333325,2.64048358730238));
#10493=CARTESIAN_POINT('Ctrl Pts',(-4.21649302087059,2.11979166666664,3.23174666634004));
#10494=CARTESIAN_POINT('Ctrl Pts',(-3.25755682958786,2.00520833333337,4.22758561320685));
#10495=CARTESIAN_POINT('Ctrl Pts',(-2.67747889815098,1.94791666666658,4.63174225660692));
#10496=CARTESIAN_POINT('Ctrl Pts',(-1.40147340323737,1.83333333333343,5.18852518461089));
#10497=CARTESIAN_POINT('Ctrl Pts',(-0.706033031254986,1.77604166666627,
5.34089658042353));
#10498=CARTESIAN_POINT('Ctrl Pts',(0.695626137060878,1.66145833333374,5.36699076915345));
#10499=CARTESIAN_POINT('Ctrl Pts',(1.40129346391331,1.60416666666663,5.24066451563091));
#10500=CARTESIAN_POINT('Ctrl Pts',(2.71521640332806,1.48958333333338,4.7246639605727));
#10501=CARTESIAN_POINT('Ctrl Pts',(3.32294022464786,1.43229166666683,4.33515684667557));
#10502=CARTESIAN_POINT('Ctrl Pts',(4.34624943902881,1.31770833333318,3.34875038791256));
#10503=CARTESIAN_POINT('Ctrl Pts',(4.76140479878007,1.26041666666641,2.75221171416214));
#10504=CARTESIAN_POINT('Ctrl Pts',(5.3330545284475,1.1458333333336,1.44031458510402));
#10505=CARTESIAN_POINT('Ctrl Pts',(5.48928815981245,1.08854166666688,0.72545744367903));
#10506=CARTESIAN_POINT('Ctrl Pts',(5.51538234856494,0.973958333333134,-0.715050549484959));
#10507=CARTESIAN_POINT('Ctrl Pts',(5.38519385944284,0.916666666666909,-1.44013464577813));
#10508=CARTESIAN_POINT('Ctrl Pts',(4.85432650277048,0.8020833333331,-2.7899492193412));
#10509=CARTESIAN_POINT('Ctrl Pts',(4.4538206724838,0.744791666666392,-3.4141337829535));
#10510=CARTESIAN_POINT('Ctrl Pts',(3.43994394623404,0.630208333333619,-4.46491326485293));
#10511=CARTESIAN_POINT('Ctrl Pts',(2.82694453016243,0.572916666666411,-4.89106734095877));
#10512=CARTESIAN_POINT('Ctrl Pts',(1.47915576698159,0.4583333333336,-5.47758387227856));
#10513=CARTESIAN_POINT('Ctrl Pts',(0.744881856102772,0.401041666666677,
-5.63767973920226));
#10514=CARTESIAN_POINT('Ctrl Pts',(-0.73447496190878,0.286458333333334,
-5.66377392797554));
#10515=CARTESIAN_POINT('Ctrl Pts',(-1.4789758276525,0.229166666666838,-5.52972320325324));
#10516=CARTESIAN_POINT('Ctrl Pts',(-2.86468203534475,0.114583333333173,
-4.9839890449698));
#10517=CARTESIAN_POINT('Ctrl Pts',(-3.50532733285514,0.0572916666665569,
-4.5724845058884));
#10518=CARTESIAN_POINT('Ctrl Pts',(-4.04445221596811,5.20417042793042E-15,
-4.05181100142375));
#10519=CARTESIAN_POINT('Origin',(-3.92444263558561,5.20417042793042E-15,
-3.92444263558507));
#10520=CARTESIAN_POINT('Origin',(-3.92444263558561,5.20417042793042E-15,
-3.92444263558507));
#10539=UNCERTAINTY_MEASURE_WITH_UNIT(LENGTH_MEASURE(0.01),#10552,
'DISTANCE_ACCURACY_VALUE',
'Maximum model space distance between geometric entities at asserted c
onnectivities');
#10540=UNCERTAINTY_MEASURE_WITH_UNIT(LENGTH_MEASURE(0.01),#10552,
'DISTANCE_ACCURACY_VALUE',
'Maximum model space distance between geometric entities at asserted c
onnectivities');
#10550=(
GEOMETRIC_REPRESENTATION_CONTEXT(3)
GLOBAL_UNCERTAINTY_ASSIGNED_CONTEXT((#10539))
GLOBAL_UNIT_ASSIGNED_CONTEXT((#10552,#10554,#10555))
REPRESENTATION_CONTEXT('','3D')
);
#10551=(
GEOMETRIC_REPRESENTATION_CONTEXT(3)
GLOBAL_UNCERTAINTY_ASSIGNED_CONTEXT((#10540))
GLOBAL_UNIT_ASSIGNED_CONTEXT((#10552,#10554,#10555))
REPRESENTATION_CONTEXT('','3D')
);
#10552=(
LENGTH_UNIT()
NAMED_UNIT(*)
SI_UNIT(.MILLI.,.METRE.)
);
#10554=(
NAMED_UNIT(*)
PLANE_ANGLE_UNIT()
SI_UNIT($,.RADIAN.)
);
#10555=(
NAMED_UNIT(*)
SI_UNIT($,.STERADIAN.)
SOLID_ANGLE_UNIT()
);
#10565=SHAPE_DEFINITION_REPRESENTATION(#10575,#10594);
#10575=PRODUCT_DEFINITION_SHAPE('',$,#10605);
#10594=SHAPE_REPRESENTATION('',(#4016),#10550);
#10595=PRODUCT_DEFINITION_CONTEXT('part definition',#10627,'design');
#10605=PRODUCT_DEFINITION('spring','Spring',#10615,#10595);
#10615=PRODUCT_DEFINITION_FORMATION('',$,#10638);
#10627=APPLICATION_CONTEXT(
'Core Data for Automotive Mechanical Design Process');
#10628=PRODUCT_CONTEXT('part definition',#10627,'mechanical');
#10638=PRODUCT('spring','Spring',$,(#10628));
#10645=PRESENTATION_STYLE_ASSIGNMENT((#10652));
#10652=SURFACE_STYLE_USAGE(.BOTH.,#10659);
#10659=SURFACE_SIDE_STYLE('',(#10666));
#10666=SURFACE_STYLE_FILL_AREA(#10673);
#10673=FILL_AREA_STYLE('Opaque(122,133,145)',(#10680));
#10680=FILL_AREA_STYLE_COLOUR('Opaque(122,133,145)',#10687);
#10687=COLOUR_RGB('Opaque(122,133,145)',0.47843137254902,0.52156862745098,
0.568627450980392);
ENDSEC;
END-ISO-10303-21;
